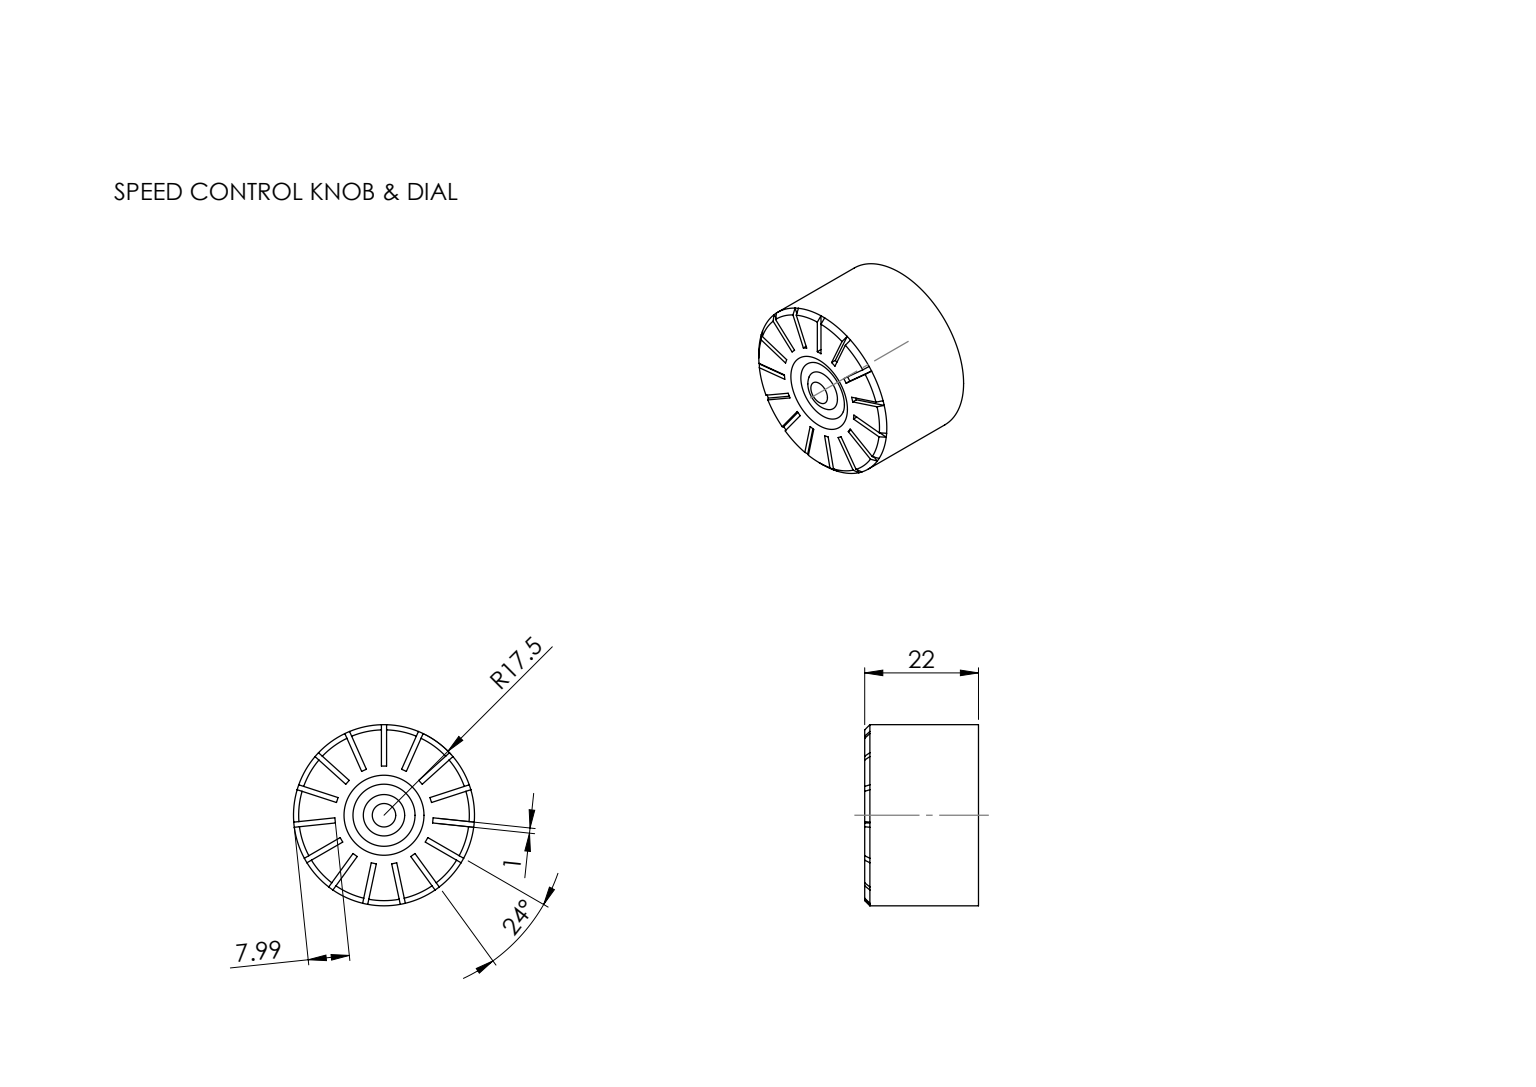
ISO-10303-21;
HEADER;
FILE_DESCRIPTION (('STEP AP214'),
    '1' );
FILE_NAME ('Speed Control Knob & Dial.step',
    '2026-10-09T15:02:13',
    ( '' ),
    ( '' ),
    'SwSTEP 2.0',
    'SolidWorks 2026',
    '' );
FILE_SCHEMA (( 'AUTOMOTIVE_DESIGN' ));
ENDSEC;

DATA;
#2=ORIENTED_EDGE ( 'NONE', *, *, #5817, .T. ) ;
#7=CARTESIAN_POINT ( 'NONE',  ( 9.881733417930924190, 8.048309972292271297, 101.0000000000000000 ) ) ;
#20=EDGE_LOOP ( 'NONE', ( #5130, #12789, #9074, #13639 ) ) ;
#24=ORIENTED_EDGE ( 'NONE', *, *, #13474, .T. ) ;
#44=DIRECTION ( 'NONE',  ( 0.000000000000000000, -0.000000000000000000, 1.000000000000000000 ) ) ;
#50=LINE ( 'NONE', #11218, #7284 ) ;
#57=ORIENTED_EDGE ( 'NONE', *, *, #15029, .T. ) ;
#62=CARTESIAN_POINT ( 'NONE',  ( -16.78599477205477797, 21.23847499609123801, 101.6666710451724214 ) ) ;
#64=CARTESIAN_POINT ( 'NONE',  ( 0.000000000000000000, 22.50000000000000000, 101.0000000000000000 ) ) ;
#65=DIRECTION ( 'NONE',  ( 0.9945218953682730678, 0.1045284632676572317, 0.000000000000000000 ) ) ;
#67=VECTOR ( 'NONE', #6603, 999.9999999999998863 ) ;
#77=ORIENTED_EDGE ( 'NONE', *, *, #283, .F. ) ;
#107=CARTESIAN_POINT ( 'NONE',  ( 0.000000000000000000, 22.50000000000000000, 102.0000000000000142 ) ) ;
#110=LINE ( 'NONE', #6455, #15051 ) ;
#112=EDGE_CURVE ( 'NONE', #12675, #13582, #5642, .T. ) ;
#127=EDGE_CURVE ( 'NONE', #6081, #8153, #2564, .T. ) ;
#131=DIRECTION ( 'NONE',  ( 0.000000000000000000, 0.000000000000000000, -1.000000000000000000 ) ) ;
#137=DIRECTION ( 'NONE',  ( 0.5000000000000039968, -0.8660254037844363761, 0.000000000000000000 ) ) ;
#142=ADVANCED_FACE ( 'NONE', ( #11706 ), #1477, .T. ) ;
#144=PLANE ( 'NONE',  #9294 ) ;
#148=PLANE ( 'NONE',  #13952 ) ;
#150=AXIS2_PLACEMENT_3D ( 'NONE', #12776, #1296, #13929 ) ;
#153=FACE_OUTER_BOUND ( 'NONE', #12318, .T. ) ;
#154=SURFACE_SIDE_STYLE ('',( #7731 ) ) ;
#162=ORIENTED_EDGE ( 'NONE', *, *, #15184, .T. ) ;
#165=ORIENTED_EDGE ( 'NONE', *, *, #12600, .T. ) ;
#166=VECTOR ( 'NONE', #9002, 1000.000000000000000 ) ;
#174=CARTESIAN_POINT ( 'NONE',  ( 14.53285685708578256, 14.68680145065703080, 102.0000000000000142 ) ) ;
#178=CIRCLE ( 'NONE', #9484, 17.50000000000000000 ) ;
#180=CARTESIAN_POINT ( 'NONE',  ( -9.189545401991425777, 24.96013318841439599, 102.0000000000000142 ) ) ;
#189=ORIENTED_EDGE ( 'NONE', *, *, #1369, .F. ) ;
#193=CARTESIAN_POINT ( 'NONE',  ( 0.000000000000000000, 22.50000000000000000, 102.0000000000000142 ) ) ;
#195=DIRECTION ( 'NONE',  ( -0.4067366430758010409, 0.9135454576426005335, 0.000000000000000000 ) ) ;
#210=EDGE_CURVE ( 'NONE', #11778, #8192, #3075, .T. ) ;
#212=CARTESIAN_POINT ( 'NONE',  ( 0.000000000000000000, 22.50000000000000000, 101.0000000000000000 ) ) ;
#224=ORIENTED_EDGE ( 'NONE', *, *, #8585, .T. ) ;
#236=PLANE ( 'NONE',  #13502 ) ;
#238=DIRECTION ( 'NONE',  ( -0.9510565162951503115, -0.3090169943749574988, 0.000000000000000000 ) ) ;
#254=CARTESIAN_POINT ( 'NONE',  ( -15.39925740754308059, 14.18658485962419569, 101.0000000000000000 ) ) ;
#264=ORIENTED_EDGE ( 'NONE', *, *, #127, .F. ) ;
#269=B_SPLINE_CURVE_WITH_KNOTS ( 'NONE', 3,
 ( #12649, #12562, #8736, #2338 ),
 .UNSPECIFIED., .F., .F.,
 ( 4, 4 ),
 ( 2.829004760667786001E-07, 0.001414802801989366570 ),
 .UNSPECIFIED. ) ;
#281=EDGE_CURVE ( 'NONE', #5931, #2031, #269, .T. ) ;
#283=EDGE_CURVE ( 'NONE', #13340, #691, #14944, .T. ) ;
#286=VERTEX_POINT ( 'NONE', #8651 ) ;
#289=FACE_OUTER_BOUND ( 'NONE', #4833, .T. ) ;
#301=DIRECTION ( 'NONE',  ( 0.9945218953682730678, 0.1045284632676572456, 0.000000000000000000 ) ) ;
#307=EDGE_CURVE ( 'NONE', #2544, #15408, #9753, .T. ) ;
#309=FACE_OUTER_BOUND ( 'NONE', #6282, .T. ) ;
#310=CARTESIAN_POINT ( 'NONE',  ( 0.000000000000000000, 22.50000000000000000, 102.0000000000000142 ) ) ;
#313=DIRECTION ( 'NONE',  ( 0.000000000000000000, 0.000000000000000000, 1.000000000000000000 ) ) ;
#322=CARTESIAN_POINT ( 'NONE',  ( -6.522576737113937817, 38.37924387995715847, 101.3333374614808662 ) ) ;
#323=ORIENTED_EDGE ( 'NONE', *, *, #16173, .F. ) ;
#325=ORIENTED_EDGE ( 'NONE', *, *, #9057, .T. ) ;
#328=CARTESIAN_POINT ( 'NONE',  ( 4.127528389677815213, 5.486372832567310454, 102.0000000000000142 ) ) ;
#337=DIRECTION ( 'NONE',  ( 1.000000000000000000, 0.000000000000000000, 0.000000000000000000 ) ) ;
#338=DIRECTION ( 'NONE',  ( 1.000000000000000000, 3.291018251567428497E-14, 0.000000000000000000 ) ) ;
#340=ADVANCED_FACE ( 'NONE', ( #12408 ), #9995, .T. ) ;
#342=DIRECTION ( 'NONE',  ( 0.000000000000000000, -0.000000000000000000, 1.000000000000000000 ) ) ;
#345=AXIS2_PLACEMENT_3D ( 'NONE', #4776, #4685, #917 ) ;
#364=ORIENTED_EDGE ( 'NONE', *, *, #5866, .F. ) ;
#367=PLANE ( 'NONE',  #5230 ) ;
#385=AXIS2_PLACEMENT_3D ( 'NONE', #4470, #15603, #705 ) ;
#387=LINE ( 'NONE', #5491, #7888 ) ;
#398=AXIS2_PLACEMENT_3D ( 'NONE', #3986, #3822, #7478 ) ;
#399=EDGE_CURVE ( 'NONE', #4332, #7924, #11576, .T. ) ;
#404=VERTEX_POINT ( 'NONE', #14726 ) ;
#413=AXIS2_PLACEMENT_3D ( 'NONE', #15842, #2171, #16155 ) ;
#414=ORIENTED_EDGE ( 'NONE', *, *, #3877, .F. ) ;
#433=ORIENTED_EDGE ( 'NONE', *, *, #9568, .T. ) ;
#446=DIRECTION ( 'NONE',  ( 0.1045284632676572456, -0.9945218953682730678, -0.000000000000000000 ) ) ;
#462=DIRECTION ( 'NONE',  ( 1.000000000000000000, 0.000000000000000000, 0.000000000000000000 ) ) ;
#474=DIRECTION ( 'NONE',  ( -0.000000000000000000, -0.000000000000000000, 1.000000000000000000 ) ) ;
#479=VECTOR ( 'NONE', #830, 1000.000000000000000 ) ;
#485=PLANE ( 'NONE',  #8421 ) ;
#502=DIRECTION ( 'NONE',  ( -0.8660254037844433705, 0.4999999999999918399, 0.000000000000000000 ) ) ;
#518=ADVANCED_FACE ( 'NONE', ( #4613 ), #3612, .F. ) ;
#544=DIRECTION ( 'NONE',  ( 1.000000000000000000, 0.000000000000000000, 0.000000000000000000 ) ) ;
#549=ORIENTED_EDGE ( 'NONE', *, *, #13824, .F. ) ;
#557=LINE ( 'NONE', #12035, #8938 ) ;
#562=VERTEX_POINT ( 'NONE', #6435 ) ;
#566=VERTEX_POINT ( 'NONE', #11495 ) ;
#569=CARTESIAN_POINT ( 'NONE',  ( 4.000000000000001776, 22.50000000000000000, 101.0000000000000000 ) ) ;
#574=DIRECTION ( 'NONE',  ( 0.000000000000000000, 0.000000000000000000, -1.000000000000000000 ) ) ;
#579=LINE ( 'NONE', #1757, #15758 ) ;
#589=VERTEX_POINT ( 'NONE', #13983 ) ;
#597=CARTESIAN_POINT ( 'NONE',  ( -8.477241335952138357, 18.18301270189218855, 101.0000000000000000 ) ) ;
#605=VERTEX_POINT ( 'NONE', #11575 ) ;
#629=AXIS2_PLACEMENT_3D ( 'NONE', #8397, #13467, #15658 ) ;
#637=CARTESIAN_POINT ( 'NONE',  ( -7.574663982647817484, 38.28367718720760138, 102.0000000000000142 ) ) ;
#646=VERTEX_POINT ( 'NONE', #3935 ) ;
#652=CARTESIAN_POINT ( 'NONE',  ( -4.056709942754369358, 5.819547430268732668, 101.3333374614808662 ) ) ;
#674=B_SPLINE_CURVE_WITH_KNOTS ( 'NONE', 3,
 ( #4274, #1766, #9418, #9340 ),
 .UNSPECIFIED., .F., .F.,
 ( 4, 4 ),
 ( 2.829004760702349710E-07, 0.001414802801989369606 ),
 .UNSPECIFIED. ) ;
#682=CARTESIAN_POINT ( 'NONE',  ( -9.877534094663211306, 8.054089844915763408, 101.0000000000000000 ) ) ;
#691=VERTEX_POINT ( 'NONE', #7507 ) ;
#694=EDGE_LOOP ( 'NONE', ( #5052, #10178, #10771, #9327 ) ) ;
#702=CARTESIAN_POINT ( 'NONE',  ( -4.127528389677584286, 5.486372832567261604, 101.0000000000000000 ) ) ;
#705=DIRECTION ( 'NONE',  ( 1.000000000000000000, 0.000000000000000000, -0.000000000000000000 ) ) ;
#707=VECTOR ( 'NONE', #13794, 1000.000000000000227 ) ;
#711=EDGE_CURVE ( 'NONE', #14691, #4152, #10547, .T. ) ;
#717=ORIENTED_EDGE ( 'NONE', *, *, #6005, .F. ) ;
#719=ORIENTED_EDGE ( 'NONE', *, *, #2125, .T. ) ;
#724=CARTESIAN_POINT ( 'NONE',  ( -4.126043002969710827, 5.493361027597350343, 101.0000000000000000 ) ) ;
#729=DIRECTION ( 'NONE',  ( -0.000000000000000000, -0.000000000000000000, 1.000000000000000000 ) ) ;
#731=CARTESIAN_POINT ( 'NONE',  ( 6.661118525004998681, 38.69041383028350367, 102.0000000000000142 ) ) ;
#734=FACE_OUTER_BOUND ( 'NONE', #14301, .T. ) ;
#739=ORIENTED_EDGE ( 'NONE', *, *, #10784, .T. ) ;
#742=LINE ( 'NONE', #7236, #3369 ) ;
#744=ORIENTED_EDGE ( 'NONE', *, *, #13835, .F. ) ;
#760=EDGE_CURVE ( 'NONE', #1819, #7317, #14134, .T. ) ;
#769=CARTESIAN_POINT ( 'NONE',  ( 0.000000000000000000, 22.50000000000000000, 101.0000000000000000 ) ) ;
#778=ORIENTED_EDGE ( 'NONE', *, *, #1765, .T. ) ;
#792=LINE ( 'NONE', #5882, #7783 ) ;
#793=VERTEX_POINT ( 'NONE', #6609 ) ;
#794=EDGE_CURVE ( 'NONE', #9739, #6366, #6691, .T. ) ;
#797=ORIENTED_EDGE ( 'NONE', *, *, #14711, .F. ) ;
#800=EDGE_CURVE ( 'NONE', #6081, #8593, #7999, .T. ) ;
#818=ORIENTED_EDGE ( 'NONE', *, *, #5743, .T. ) ;
#828=DIRECTION ( 'NONE',  ( 1.000000000000000000, -5.352861011585576290E-15, 0.000000000000000000 ) ) ;
#830=DIRECTION ( 'NONE',  ( -0.000000000000000000, -0.000000000000000000, 1.000000000000000000 ) ) ;
#833=LINE ( 'NONE', #15967, #10244 ) ;
#836=CARTESIAN_POINT ( 'NONE',  ( 0.000000000000000000, 22.50000000000000000, 80.00000000000000000 ) ) ;
#845=DIRECTION ( 'NONE',  ( -0.9135454576426004225, -0.4067366430758009854, 0.000000000000000000 ) ) ;
#860=VERTEX_POINT ( 'NONE', #11908 ) ;
#874=CARTESIAN_POINT ( 'NONE',  ( 3.407225380398686276, 31.38205016914263723, 102.0000000000000142 ) ) ;
#875=ORIENTED_EDGE ( 'NONE', *, *, #8946, .T. ) ;
#878=DIRECTION ( 'NONE',  ( 0.8660254037844363761, 0.5000000000000041078, 0.000000000000000000 ) ) ;
#888=CARTESIAN_POINT ( 'NONE',  ( -6.661118525005218949, 38.69041383028340420, 102.0000000000000142 ) ) ;
#889=DIRECTION ( 'NONE',  ( -0.000000000000000000, -0.000000000000000000, 1.000000000000000000 ) ) ;
#890=DIRECTION ( 'NONE',  ( 0.000000000000000000, 0.000000000000000000, -1.000000000000000000 ) ) ;
#895=VERTEX_POINT ( 'NONE', #1676 ) ;
#900=ORIENTED_EDGE ( 'NONE', *, *, #11699, .F. ) ;
#915=EDGE_CURVE ( 'NONE', #9440, #646, #6307, .T. ) ;
#917=DIRECTION ( 'NONE',  ( 1.000000000000000000, 0.000000000000000000, 0.000000000000000000 ) ) ;
#918=ORIENTED_EDGE ( 'NONE', *, *, #1112, .T. ) ;
#919=DIRECTION ( 'NONE',  ( -0.000000000000000000, 0.000000000000000000, 1.000000000000000000 ) ) ;
#925=DIRECTION ( 'NONE',  ( -0.000000000000000000, -0.000000000000000000, -1.000000000000000000 ) ) ;
#926=LINE ( 'NONE', #8666, #14148 ) ;
#927=DIRECTION ( 'NONE',  ( 0.000000000000000000, 0.000000000000000000, 1.000000000000000000 ) ) ;
#941=ORIENTED_EDGE ( 'NONE', *, *, #4990, .F. ) ;
#956=VECTOR ( 'NONE', #12319, 1000.000000000000000 ) ;
#959=ORIENTED_EDGE ( 'NONE', *, *, #281, .F. ) ;
#960=VERTEX_POINT ( 'NONE', #8246 ) ;
#977=ORIENTED_EDGE ( 'NONE', *, *, #9370, .T. ) ;
#987=( NAMED_UNIT ( * ) PLANE_ANGLE_UNIT ( ) SI_UNIT ( $, .RADIAN. ) );
#989=CARTESIAN_POINT ( 'NONE',  ( -16.16503364901097939, 28.27806893495044349, 101.3333374614808662 ) ) ;
#996=CARTESIAN_POINT ( 'NONE',  ( 0.000000000000000000, 22.50000000000000000, 101.0000000000000000 ) ) ;
#1002=EDGE_CURVE ( 'NONE', #11153, #15748, #13312, .T. ) ;
#1005=LINE ( 'NONE', #8661, #11852 ) ;
#1007=CARTESIAN_POINT ( 'NONE',  ( 14.61046079763427130, 13.48729625631194118, 101.3333374614808662 ) ) ;
#1033=ADVANCED_FACE ( 'NONE', ( #14549 ), #10907, .F. ) ;
#1037=ADVANCED_FACE ( 'NONE', ( #12061 ), #4680, .T. ) ;
#1040=EDGE_LOOP ( 'NONE', ( #13375, #11613, #1901, #5104 ) ) ;
#1041=ORIENTED_EDGE ( 'NONE', *, *, #14423, .T. ) ;
#1044=LINE ( 'NONE', #12452, #15798 ) ;
#1047=CIRCLE ( 'NONE', #1583, 2.267949192431125027 ) ;
#1052=CARTESIAN_POINT ( 'NONE',  ( -15.53071739328007794, 28.07196708982276334, 102.0000000000000142 ) ) ;
#1054=FACE_OUTER_BOUND ( 'NONE', #13700, .T. ) ;
#1057=EDGE_LOOP ( 'NONE', ( #1893, #7443, #15977, #14426 ) ) ;
#1083=VERTEX_POINT ( 'NONE', #4517 ) ;
#1085=ORIENTED_EDGE ( 'NONE', *, *, #15147, .F. ) ;
#1086=DIRECTION ( 'NONE',  ( -0.8660254037844433705, 0.4999999999999918954, 0.000000000000000000 ) ) ;
#1094=PLANE ( 'NONE',  #12119 ) ;
#1100=EDGE_CURVE ( 'NONE', #1499, #2544, #12417, .T. ) ;
#1101=VERTEX_POINT ( 'NONE', #7092 ) ;
#1109=ADVANCED_FACE ( 'NONE', ( #13477 ), #12152, .T. ) ;
#1112=EDGE_CURVE ( 'NONE', #860, #7211, #5048, .T. ) ;
#1115=ADVANCED_FACE ( 'NONE', ( #1155 ), #12485, .T. ) ;
#1118=ORIENTED_EDGE ( 'NONE', *, *, #15652, .T. ) ;
#1123=CARTESIAN_POINT ( 'NONE',  ( 17.44929222242216227, 21.16875962481693207, 101.0000000000000000 ) ) ;
#1125=DIRECTION ( 'NONE',  ( 0.000000000000000000, 0.000000000000000000, -1.000000000000000000 ) ) ;
#1130=CARTESIAN_POINT ( 'NONE',  ( 4.320770838041294581, 30.97531352606685218, 101.0000000000000000 ) ) ;
#1134=ORIENTED_EDGE ( 'NONE', *, *, #1002, .F. ) ;
#1139=ADVANCED_FACE ( 'NONE', ( #16220 ), #10024, .T. ) ;
#1141=LINE ( 'NONE', #8801, #3640 ) ;
#1145=ORIENTED_EDGE ( 'NONE', *, *, #1475, .F. ) ;
#1148=CARTESIAN_POINT ( 'NONE',  ( 0.000000000000000000, 22.50000000000000000, 102.0000000000000142 ) ) ;
#1151=DIRECTION ( 'NONE',  ( 0.8660254037844432595, -0.4999999999999920064, 0.000000000000000000 ) ) ;
#1155=FACE_OUTER_BOUND ( 'NONE', #4460, .T. ) ;
#1161=EDGE_LOOP ( 'NONE', ( #1118, #2203, #12678, #13882 ) ) ;
#1168=DIRECTION ( 'NONE',  ( 0.000000000000000000, 0.000000000000000000, -1.000000000000000000 ) ) ;
#1182=AXIS2_PLACEMENT_3D ( 'NONE', #5912, #10972, #15193 ) ;
#1200=ORIENTED_EDGE ( 'NONE', *, *, #13732, .F. ) ;
#1201=AXIS2_PLACEMENT_3D ( 'NONE', #11274, #16332, #1361 ) ;
#1208=CARTESIAN_POINT ( 'NONE',  ( 1.486087262401875941, 13.10364194761998213, 101.0000000000000000 ) ) ;
#1218=DIRECTION ( 'NONE',  ( 0.000000000000000000, 0.000000000000000000, -1.000000000000000000 ) ) ;
#1219=CIRCLE ( 'NONE', #2556, 16.50000000000000711 ) ;
#1221=EDGE_CURVE ( 'NONE', #14428, #404, #5255, .T. ) ;
#1233=AXIS2_PLACEMENT_3D ( 'NONE', #15547, #11894, #4178 ) ;
#1237=CARTESIAN_POINT ( 'NONE',  ( 0.000000000000000000, 22.50000000000000000, 102.0000000000000142 ) ) ;
#1239=CARTESIAN_POINT ( 'NONE',  ( 0.000000000000000000, 22.50000000000000000, 102.0000000000000142 ) ) ;
#1246=DIRECTION ( 'NONE',  ( 0.000000000000000000, 0.000000000000000000, -1.000000000000000000 ) ) ;
#1249=EDGE_LOOP ( 'NONE', ( #3388, #224, #10891, #15269 ) ) ;
#1250=EDGE_CURVE ( 'NONE', #9378, #8439, #5819, .T. ) ;
#1251=CARTESIAN_POINT ( 'NONE',  ( 0.000000000000000000, 22.50000000000000000, 101.0000000000000000 ) ) ;
#1252=ORIENTED_EDGE ( 'NONE', *, *, #15652, .F. ) ;
#1262=LINE ( 'NONE', #8827, #166 ) ;
#1264=DIRECTION ( 'NONE',  ( 1.000000000000000000, 0.000000000000000000, 0.000000000000000000 ) ) ;
#1266=CARTESIAN_POINT ( 'NONE',  ( 0.000000000000000000, 22.50000000000000000, 101.0000000000000000 ) ) ;
#1271=EDGE_CURVE ( 'NONE', #1479, #2396, #6753, .T. ) ;
#1276=ORIENTED_EDGE ( 'NONE', *, *, #15012, .T. ) ;
#1291=EDGE_LOOP ( 'NONE', ( #5186, #12830, #15543, #6502 ) ) ;
#1296=DIRECTION ( 'NONE',  ( 0.000000000000000000, 0.000000000000000000, -1.000000000000000000 ) ) ;
#1305=ORIENTED_EDGE ( 'NONE', *, *, #14153, .F. ) ;
#1310=ORIENTED_EDGE ( 'NONE', *, *, #14892, .T. ) ;
#1319=CARTESIAN_POINT ( 'NONE',  ( 7.394441145214595501, 28.48516834767053751, 101.0000000000000000 ) ) ;
#1326=VERTEX_POINT ( 'NONE', #11799 ) ;
#1331=CARTESIAN_POINT ( 'NONE',  ( -4.127528389677584286, 5.486372832567261604, 101.0000000000000000 ) ) ;
#1336=CARTESIAN_POINT ( 'NONE',  ( -10.69075041230567891, 8.636095224584611429, 101.0000000000000000 ) ) ;
#1354=EDGE_CURVE ( 'NONE', #13340, #7372, #2628, .T. ) ;
#1361=DIRECTION ( 'NONE',  ( -1.000000000000000000, 0.000000000000000000, 0.000000000000000000 ) ) ;
#1369=EDGE_CURVE ( 'NONE', #9016, #14108, #178, .T. ) ;
#1372=ORIENTED_EDGE ( 'NONE', *, *, #7951, .F. ) ;
#1376=ADVANCED_FACE ( 'NONE', ( #9478 ), #8468, .F. ) ;
#1384=LINE ( 'NONE', #16276, #6059 ) ;
#1389=ORIENTED_EDGE ( 'NONE', *, *, #1354, .F. ) ;
#1393=DIRECTION ( 'NONE',  ( -0.3090169943749573878, 0.9510565162951503115, 0.000000000000000000 ) ) ;
#1396=DIRECTION ( 'NONE',  ( -0.7431448254773861395, -0.6691306063588672304, 0.000000000000000000 ) ) ;
#1398=DIRECTION ( 'NONE',  ( 0.8090169943749504489, -0.5877852522924689183, 0.000000000000000000 ) ) ;
#1404=CARTESIAN_POINT ( 'NONE',  ( 1.486087262401875941, 13.10364194761998213, 101.0000000000000000 ) ) ;
#1412=CARTESIAN_POINT ( 'NONE',  ( 0.000000000000000000, 22.50000000000000000, 102.0000000000000142 ) ) ;
#1433=ORIENTED_EDGE ( 'NONE', *, *, #15400, .T. ) ;
#1451=AXIS2_PLACEMENT_3D ( 'NONE', #6325, #11391, #3740 ) ;
#1458=VECTOR ( 'NONE', #4886, 999.9999999999998863 ) ;
#1466=LINE ( 'NONE', #4050, #4788 ) ;
#1470=DIRECTION ( 'NONE',  ( 1.224646799147353207E-16, 1.000000000000000000, -0.000000000000000000 ) ) ;
#1475=EDGE_CURVE ( 'NONE', #14428, #7907, #7062, .T. ) ;
#1476=ORIENTED_EDGE ( 'NONE', *, *, #12004, .T. ) ;
#1477=PLANE ( 'NONE',  #14226 ) ;
#1479=VERTEX_POINT ( 'NONE', #8774 ) ;
#1482=CARTESIAN_POINT ( 'NONE',  ( 7.300484685132999196, 37.66786040234666189, 101.6666710451724214 ) ) ;
#1485=VECTOR ( 'NONE', #16302, 1000.000000000000000 ) ;
#1487=AXIS2_PLACEMENT_3D ( 'NONE', #7913, #11658, #14139 ) ;
#1495=DIRECTION ( 'NONE',  ( -0.3090169943749574988, 0.9510565162951503115, 0.000000000000000000 ) ) ;
#1497=CARTESIAN_POINT ( 'NONE',  ( 15.83973438765496056, 27.12091057352781931, 102.0000000000000142 ) ) ;
#1499=VERTEX_POINT ( 'NONE', #14772 ) ;
#1511=LINE ( 'NONE', #10413, #67 ) ;
#1515=VECTOR ( 'NONE', #9722, 1000.000000000000000 ) ;
#1524=ADVANCED_FACE ( 'NONE', ( #5735 ), #9807, .T. ) ;
#1527=EDGE_CURVE ( 'NONE', #3819, #3901, #12127, .T. ) ;
#1533=B_SPLINE_CURVE_WITH_KNOTS ( 'NONE', 3,
 ( #5559, #2707, #9037, #14261 ),
 .UNSPECIFIED., .F., .F.,
 ( 4, 4 ),
 ( 2.829004760673920638E-07, 0.001414802801989365486 ),
 .UNSPECIFIED. ) ;
#1537=LINE ( 'NONE', #6373, #11863 ) ;
#1547=ORIENTED_EDGE ( 'NONE', *, *, #15147, .T. ) ;
#1548=CARTESIAN_POINT ( 'NONE',  ( -13.22516817658079624, 40.70288237343621063, 101.0000000000000000 ) ) ;
#1550=CARTESIAN_POINT ( 'NONE',  ( -14.82166083077704499, 14.52006039870307852, 101.6666710451724214 ) ) ;
#1558=FACE_OUTER_BOUND ( 'NONE', #10631, .T. ) ;
#1561=ORIENTED_EDGE ( 'NONE', *, *, #11744, .T. ) ;
#1562=CARTESIAN_POINT ( 'NONE',  ( -0.5000000000000000000, 39.65938208326293335, 101.3333374618097480 ) ) ;
#1563=EDGE_LOOP ( 'NONE', ( #13749, #13457, #3721, #959 ) ) ;
#1564=ORIENTED_EDGE ( 'NONE', *, *, #1250, .T. ) ;
#1570=VECTOR ( 'NONE', #9716, 1000.000000000000114 ) ;
#1573=DIRECTION ( 'NONE',  ( -0.000000000000000000, -0.000000000000000000, 1.000000000000000000 ) ) ;
#1583=AXIS2_PLACEMENT_3D ( 'NONE', #310, #15194, #13947 ) ;
#1584=ORIENTED_EDGE ( 'NONE', *, *, #1798, .F. ) ;
#1593=CARTESIAN_POINT ( 'NONE',  ( 0.000000000000000000, 22.50000000000000000, 102.0000000000000142 ) ) ;
#1601=FACE_OUTER_BOUND ( 'NONE', #8159, .T. ) ;
#1622=EDGE_LOOP ( 'NONE', ( #5422, #797, #7323, #9730 ) ) ;
#1635=CARTESIAN_POINT ( 'NONE',  ( -6.725310538855818976, 29.22831317314782851, 101.0000000000000000 ) ) ;
#1636=ORIENTED_EDGE ( 'NONE', *, *, #16217, .T. ) ;
#1641=VERTEX_POINT ( 'NONE', #2989 ) ;
#1656=FACE_OUTER_BOUND ( 'NONE', #3657, .T. ) ;
#1660=ORIENTED_EDGE ( 'NONE', *, *, #5200, .T. ) ;
#1662=ADVANCED_FACE ( 'NONE', ( #1656 ), #485, .T. ) ;
#1674=CARTESIAN_POINT ( 'NONE',  ( 5.988468393966018155, 15.10823117958429584, 101.0000000000000000 ) ) ;
#1676=CARTESIAN_POINT ( 'NONE',  ( -2.464234863135557063, 13.31155363843772932, 102.0000000000000142 ) ) ;
#1685=ORIENTED_EDGE ( 'NONE', *, *, #6952, .T. ) ;
#1702=ORIENTED_EDGE ( 'NONE', *, *, #5817, .F. ) ;
#1705=CARTESIAN_POINT ( 'NONE',  ( -17.35186893731094671, 20.17349094513186358, 101.0000000000000000 ) ) ;
#1726=DIRECTION ( 'NONE',  ( 0.000000000000000000, 0.000000000000000000, -1.000000000000000000 ) ) ;
#1735=CIRCLE ( 'NONE', #12622, 4.000000000000001776 ) ;
#1736=DIRECTION ( 'NONE',  ( 0.5000000000000039968, -0.8660254037844363761, 0.000000000000000000 ) ) ;
#1744=AXIS2_PLACEMENT_3D ( 'NONE', #14955, #16212, #4844 ) ;
#1747=VECTOR ( 'NONE', #4128, 1000.000000000000000 ) ;
#1757=CARTESIAN_POINT ( 'NONE',  ( 0.5000000000000000000, 39.99999999999999289, 102.0000000000000142 ) ) ;
#1762=CIRCLE ( 'NONE', #5243, 17.50000000000000000 ) ;
#1765=EDGE_CURVE ( 'NONE', #5661, #2974, #3228, .T. ) ;
#1766=CARTESIAN_POINT ( 'NONE',  ( 13.08647130699016614, 33.61029532559867050, 101.3333374614808662 ) ) ;
#1769=VERTEX_POINT ( 'NONE', #13455 ) ;
#1770=CARTESIAN_POINT ( 'NONE',  ( 0.000000000000000000, 22.50000000000000000, 101.0000000000000000 ) ) ;
#1772=VECTOR ( 'NONE', #11819, 1000.000000000000000 ) ;
#1775=VECTOR ( 'NONE', #15211, 1000.000000000000000 ) ;
#1779=DIRECTION ( 'NONE',  ( 0.9945218953682730678, 0.1045284632676572456, 0.000000000000000000 ) ) ;
#1790=ORIENTED_EDGE ( 'NONE', *, *, #2785, .T. ) ;
#1791=LINE ( 'NONE', #13102, #1747 ) ;
#1795=DIRECTION ( 'NONE',  ( -0.7431448254773954654, 0.6691306063588569053, 0.000000000000000000 ) ) ;
#1798=EDGE_CURVE ( 'NONE', #13034, #9095, #2062, .T. ) ;
#1819=VERTEX_POINT ( 'NONE', #7313 ) ;
#1822=ORIENTED_EDGE ( 'NONE', *, *, #13766, .T. ) ;
#1826=ORIENTED_EDGE ( 'NONE', *, *, #1221, .T. ) ;
#1827=CARTESIAN_POINT ( 'NONE',  ( -10.09851121871618140, 9.451242543235633065, 102.0000000000000142 ) ) ;
#1831=ADVANCED_FACE ( 'NONE', ( #734 ), #8442, .T. ) ;
#1836=CARTESIAN_POINT ( 'NONE',  ( 3.147895402236133400, 5.285449336779636909, 101.0000000000000000 ) ) ;
#1841=EDGE_CURVE ( 'NONE', #7924, #286, #1384, .T. ) ;
#1859=ADVANCED_FACE ( 'NONE', ( #12864 ), #16446, .F. ) ;
#1864=FACE_OUTER_BOUND ( 'NONE', #13111, .T. ) ;
#1873=EDGE_CURVE ( 'NONE', #2880, #10320, #13746, .T. ) ;
#1893=ORIENTED_EDGE ( 'NONE', *, *, #1112, .F. ) ;
#1897=ORIENTED_EDGE ( 'NONE', *, *, #13064, .F. ) ;
#1901=ORIENTED_EDGE ( 'NONE', *, *, #5685, .F. ) ;
#1903=CARTESIAN_POINT ( 'NONE',  ( -3.918041248536338728, 6.471932344328960696, 102.0000000000000142 ) ) ;
#1918=UNCERTAINTY_MEASURE_WITH_UNIT (LENGTH_MEASURE( 1.000000000000000082E-05 ), #12798, 'distance_accuracy_value', 'NONE');
#1921=CARTESIAN_POINT ( 'NONE',  ( 14.90544456622775904, 13.31698729810792692, 101.0000000000000000 ) ) ;
#1929=DIRECTION ( 'NONE',  ( 0.4067366430758010964, -0.9135454576426004225, 0.000000000000000000 ) ) ;
#1932=VECTOR ( 'NONE', #15469, 999.9999999999998863 ) ;
#1944=ORIENTED_EDGE ( 'NONE', *, *, #5416, .F. ) ;
#1945=CARTESIAN_POINT ( 'NONE',  ( 3.918041248536554555, 6.471932344329013098, 102.0000000000000142 ) ) ;
#1948=CARTESIAN_POINT ( 'NONE',  ( 0.000000000000000000, 22.50000000000000000, 102.0000000000000142 ) ) ;
#1991=DIRECTION ( 'NONE',  ( 0.000000000000000000, 0.000000000000000000, -1.000000000000000000 ) ) ;
#2002=VECTOR ( 'NONE', #16137, 1000.000000000000000 ) ;
#2015=VECTOR ( 'NONE', #7830, 1000.000000000000000 ) ;
#2017=FACE_OUTER_BOUND ( 'NONE', #8126, .T. ) ;
#2031=VERTEX_POINT ( 'NONE', #12201 ) ;
#2039=VECTOR ( 'NONE', #16120, 1000.000000000000114 ) ;
#2046=ADVANCED_FACE ( 'NONE', ( #9713 ), #3396, .F. ) ;
#2060=CARTESIAN_POINT ( 'NONE',  ( 15.83973438765496056, 27.12091057352781931, 102.0000000000000142 ) ) ;
#2062=LINE ( 'NONE', #8382, #3390 ) ;
#2063=CARTESIAN_POINT ( 'NONE',  ( -7.571758127758879908, 38.27715053026740577, 101.0000000000000000 ) ) ;
#2068=ORIENTED_EDGE ( 'NONE', *, *, #7249, .T. ) ;
#2076=DIRECTION ( 'NONE',  ( 0.000000000000000000, 0.000000000000000000, -1.000000000000000000 ) ) ;
#2079=DIRECTION ( 'NONE',  ( 1.000000000000000000, 7.930164461608261426E-16, 0.000000000000000000 ) ) ;
#2088=PRODUCT_DEFINITION_CONTEXT ( 'detailed design', #14591, 'design' ) ;
#2093=FACE_OUTER_BOUND ( 'NONE', #8210, .T. ) ;
#2096=STYLED_ITEM ( 'NONE', ( #12300 ), #3320 ) ;
#2114=LINE ( 'NONE', #5876, #1458 ) ;
#2125=EDGE_CURVE ( 'NONE', #404, #7781, #14519, .T. ) ;
#2126=ORIENTED_EDGE ( 'NONE', *, *, #13766, .F. ) ;
#2140=CARTESIAN_POINT ( 'NONE',  ( -0.4999999999999990563, 31.99999999999998579, 101.0000000000000000 ) ) ;
#2146=ORIENTED_EDGE ( 'NONE', *, *, #10006, .T. ) ;
#2150=ORIENTED_EDGE ( 'NONE', *, *, #15029, .F. ) ;
#2152=DIRECTION ( 'NONE',  ( 0.5877852522924688072, 0.8090169943749505599, 0.000000000000000000 ) ) ;
#2158=CARTESIAN_POINT ( 'NONE',  ( 0.000000000000000000, 0.000000000000000000, 0.000000000000000000 ) ) ;
#2164=DIRECTION ( 'NONE',  ( 1.000000000000000000, 0.000000000000000000, 0.000000000000000000 ) ) ;
#2166=CARTESIAN_POINT ( 'NONE',  ( 9.485510086921706829, 8.593664601562213790, 101.6666710451724214 ) ) ;
#2169=LINE ( 'NONE', #12241, #956 ) ;
#2171=DIRECTION ( 'NONE',  ( -0.3090169943749448422, -0.9510565162951544194, 0.000000000000000000 ) ) ;
#2188=ORIENTED_EDGE ( 'NONE', *, *, #9653, .T. ) ;
#2203=ORIENTED_EDGE ( 'NONE', *, *, #13732, .T. ) ;
#2207=CARTESIAN_POINT ( 'NONE',  ( 12.16951863902660236, 34.13030016454095517, 101.6666710451724214 ) ) ;
#2224=VERTEX_POINT ( 'NONE', #2382 ) ;
#2229=DIRECTION ( 'NONE',  ( 0.000000000000000000, 1.000000000000000000, 0.000000000000000000 ) ) ;
#2236=CARTESIAN_POINT ( 'NONE',  ( -15.84787772126911776, 28.17501872725009093, 101.6666710451724214 ) ) ;
#2238=DIRECTION ( 'NONE',  ( 0.8090169943749426773, 0.5877852522924797984, 0.000000000000000000 ) ) ;
#2249=CARTESIAN_POINT ( 'NONE',  ( 9.681523229999685398, 8.323875655254958872, 101.3333374614808662 ) ) ;
#2253=VECTOR ( 'NONE', #11449, 1000.000000000000114 ) ;
#2254=EDGE_CURVE ( 'NONE', #7234, #12941, #8612, .T. ) ;
#2263=EDGE_CURVE ( 'NONE', #5800, #1641, #12454, .T. ) ;
#2267=AXIS2_PLACEMENT_3D ( 'NONE', #7, #12739, #12815 ) ;
#2277=VECTOR ( 'NONE', #16147, 1000.000000000000000 ) ;
#2280=CIRCLE ( 'NONE', #5231, 17.50000000000000000 ) ;
#2292=CARTESIAN_POINT ( 'NONE',  ( -8.880528407616480990, 25.91118970470954963, 101.0000000000000000 ) ) ;
#2293=ORIENTED_EDGE ( 'NONE', *, *, #6374, .T. ) ;
#2297=CARTESIAN_POINT ( 'NONE',  ( -3.407225380398804404, 31.38205016914259105, 102.0000000000000142 ) ) ;
#2301=ADVANCED_FACE ( 'NONE', ( #4900 ), #15014, .F. ) ;
#2309=CIRCLE ( 'NONE', #14787, 6.000000000000001776 ) ;
#2316=ORIENTED_EDGE ( 'NONE', *, *, #14670, .T. ) ;
#2322=DIRECTION ( 'NONE',  ( -0.000000000000000000, 0.000000000000000000, 1.000000000000000000 ) ) ;
#2323=LINE ( 'NONE', #5260, #14851 ) ;
#2325=CARTESIAN_POINT ( 'NONE',  ( -15.53071739328007794, 28.07196708982276334, 102.0000000000000142 ) ) ;
#2338=CARTESIAN_POINT ( 'NONE',  ( -14.03285685708567065, 13.82077604687239258, 102.0000000000000142 ) ) ;
#2347=CARTESIAN_POINT ( 'NONE',  ( 13.22516817658054933, 40.70288237343638826, 101.0000000000000000 ) ) ;
#2352=PLANE ( 'NONE',  #5274 ) ;
#2358=EDGE_CURVE ( 'NONE', #15408, #2396, #13233, .T. ) ;
#2375=DIRECTION ( 'NONE',  ( -0.000000000000000000, -0.000000000000000000, 1.000000000000000000 ) ) ;
#2377=ORIENTED_EDGE ( 'NONE', *, *, #14727, .T. ) ;
#2382=CARTESIAN_POINT ( 'NONE',  ( 9.189545401991395579, 24.96013318841451678, 102.0000000000000142 ) ) ;
#2391=EDGE_CURVE ( 'NONE', #3858, #9016, #6881, .T. ) ;
#2396=VERTEX_POINT ( 'NONE', #12147 ) ;
#2401=ORIENTED_EDGE ( 'NONE', *, *, #794, .T. ) ;
#2411=CARTESIAN_POINT ( 'NONE',  ( 6.251299836021209089, 37.76994598419266680, 102.0000000000000142 ) ) ;
#2416=ORIENTED_EDGE ( 'NONE', *, *, #15170, .F. ) ;
#2422=LINE ( 'NONE', #13734, #11051 ) ;
#2459=FACE_OUTER_BOUND ( 'NONE', #4151, .T. ) ;
#2467=CARTESIAN_POINT ( 'NONE',  ( -7.571758127758879908, 38.27715053026740577, 101.0000000000000000 ) ) ;
#2468=EDGE_CURVE ( 'NONE', #7372, #2224, #3246, .T. ) ;
#2471=DIRECTION ( 'NONE',  ( 1.000000000000000000, 0.000000000000000000, 0.000000000000000000 ) ) ;
#2481=VECTOR ( 'NONE', #13307, 1000.000000000000000 ) ;
#2485=DIRECTION ( 'NONE',  ( 1.000000000000000000, 0.000000000000000000, 0.000000000000000000 ) ) ;
#2488=FACE_OUTER_BOUND ( 'NONE', #20, .T. ) ;
#2492=DIRECTION ( 'NONE',  ( 0.2079116908177664202, -0.9781476007338041345, 0.000000000000000000 ) ) ;
#2505=AXIS2_PLACEMENT_3D ( 'NONE', #14076, #2691, #3785 ) ;
#2540=ORIENTED_EDGE ( 'NONE', *, *, #9370, .F. ) ;
#2544=VERTEX_POINT ( 'NONE', #13551 ) ;
#2546=LINE ( 'NONE', #2297, #2253 ) ;
#2548=CARTESIAN_POINT ( 'NONE',  ( -7.977241335952133916, 17.31698729810774751, 101.0000000000000000 ) ) ;
#2553=CIRCLE ( 'NONE', #13434, 17.50000000000000000 ) ;
#2556=AXIS2_PLACEMENT_3D ( 'NONE', #1237, #3744, #6331 ) ;
#2557=ADVANCED_FACE ( 'NONE', ( #11071 ), #4767, .T. ) ;
#2558=DIRECTION ( 'NONE',  ( -0.5877852522924797984, 0.8090169943749424553, 0.000000000000000000 ) ) ;
#2564=LINE ( 'NONE', #7643, #8117 ) ;
#2568=DIRECTION ( 'NONE',  ( 0.000000000000000000, -0.000000000000000000, -1.000000000000000000 ) ) ;
#2572=CARTESIAN_POINT ( 'NONE',  ( 0.000000000000000000, 22.50000000000000000, 101.0000000000000000 ) ) ;
#2580=DIRECTION ( 'NONE',  ( 0.9781476007338041345, 0.2079116908177664202, 0.000000000000000000 ) ) ;
#2585=ORIENTED_EDGE ( 'NONE', *, *, #16278, .T. ) ;
#2590=LINE ( 'NONE', #12895, #1775 ) ;
#2596=DIRECTION ( 'NONE',  ( -0.9945218953682744001, 0.1045284632676435205, 0.000000000000000000 ) ) ;
#2598=EDGE_CURVE ( 'NONE', #8439, #16202, #5043, .T. ) ;
#2606=AXIS2_PLACEMENT_3D ( 'NONE', #5818, #131, #5078 ) ;
#2614=FACE_OUTER_BOUND ( 'NONE', #8305, .T. ) ;
#2617=AXIS2_PLACEMENT_3D ( 'NONE', #12532, #1125, #15100 ) ;
#2628=B_SPLINE_CURVE_WITH_KNOTS ( 'NONE', 3,
 ( #2987, #8056, #2736, #1497 ),
 .UNSPECIFIED., .F., .F.,
 ( 4, 4 ),
 ( 2.829004760679149478E-07, 0.001414802801989369172 ),
 .UNSPECIFIED. ) ;
#2629=CARTESIAN_POINT ( 'NONE',  ( -12.16951863902676223, 34.13030016454078464, 101.6666710451724214 ) ) ;
#2640=ORIENTED_EDGE ( 'NONE', *, *, #9573, .F. ) ;
#2648=CARTESIAN_POINT ( 'NONE',  ( 0.5000000000000009992, 31.99999999999998579, 101.0000000000000000 ) ) ;
#2649=CARTESIAN_POINT ( 'NONE',  ( 2.464234863135679188, 13.31155363843775064, 102.0000000000000142 ) ) ;
#2651=EDGE_CURVE ( 'NONE', #15408, #1769, #15198, .T. ) ;
#2654=CARTESIAN_POINT ( 'NONE',  ( -5.988468393965924008, 15.10823117958422301, 102.0000000000000142 ) ) ;
#2655=DIRECTION ( 'NONE',  ( 0.8090169943749505599, -0.5877852522924688072, -0.000000000000000000 ) ) ;
#2660=DIRECTION ( 'NONE',  ( 0.000000000000000000, 0.000000000000000000, -1.000000000000000000 ) ) ;
#2663=CARTESIAN_POINT ( 'NONE',  ( -6.658212670116278709, 38.68388717334321569, 101.0000000000000000 ) ) ;
#2664=VERTEX_POINT ( 'NONE', #7730 ) ;
#2685=ORIENTED_EDGE ( 'NONE', *, *, #12100, .T. ) ;
#2691=DIRECTION ( 'NONE',  ( 0.9781476007338041345, 0.2079116908177665313, 0.000000000000000000 ) ) ;
#2698=ADVANCED_FACE ( 'NONE', ( #153 ), #3746, .T. ) ;
#2706=DIRECTION ( 'NONE',  ( 0.9945218953682730678, 0.1045284632676572317, 0.000000000000000000 ) ) ;
#2707=CARTESIAN_POINT ( 'NONE',  ( 15.11046079763426420, 14.35332166009638222, 101.3333374614808662 ) ) ;
#2718=AXIS2_PLACEMENT_3D ( 'NONE', #10721, #12040, #4408 ) ;
#2723=ORIENTED_EDGE ( 'NONE', *, *, #4292, .F. ) ;
#2729=DIRECTION ( 'NONE',  ( -0.000000000000000000, -0.000000000000000000, -1.000000000000000000 ) ) ;
#2733=VECTOR ( 'NONE', #7619, 1000.000000000000000 ) ;
#2736=CARTESIAN_POINT ( 'NONE',  ( 16.15689471564400037, 27.22396221095515045, 101.6666710451724214 ) ) ;
#2740=PRODUCT_DEFINITION ( 'UNKNOWN', '', #6278, #2088 ) ;
#2743=VERTEX_POINT ( 'NONE', #14364 ) ;
#2752=LINE ( 'NONE', #3085, #16275 ) ;
#2779=DIRECTION ( 'NONE',  ( -0.9945218953682744001, 0.1045284632676435205, 0.000000000000000000 ) ) ;
#2785=EDGE_CURVE ( 'NONE', #10405, #10911, #9472, .T. ) ;
#2793=CARTESIAN_POINT ( 'NONE',  ( -15.39925740754308059, 14.18658485962419569, 101.0000000000000000 ) ) ;
#2808=CARTESIAN_POINT ( 'NONE',  ( -0.5000000000000000000, 39.99285568453590400, 101.0000000000000000 ) ) ;
#2809=EDGE_LOOP ( 'NONE', ( #5254, #6057, #13537, #8063 ) ) ;
#2819=CONICAL_SURFACE ( 'NONE', #3355, 16.50000000000000711, 0.7853981633974447263 ) ;
#2826=CARTESIAN_POINT ( 'NONE',  ( -5.988468393965924008, 15.10823117958422301, 101.0000000000000000 ) ) ;
#2834=VECTOR ( 'NONE', #14855, 1000.000000000000000 ) ;
#2837=DIRECTION ( 'NONE',  ( -0.7431448254773861395, -0.6691306063588672304, 0.000000000000000000 ) ) ;
#2839=EDGE_LOOP ( 'NONE', ( #1252, #10363, #14918, #2723 ) ) ;
#2850=VECTOR ( 'NONE', #5336, 1000.000000000000000 ) ;
#2855=LINE ( 'NONE', #9172, #10962 ) ;
#2856=ORIENTED_EDGE ( 'NONE', *, *, #11284, .F. ) ;
#2857=ADVANCED_FACE ( 'NONE', ( #9140 ), #236, .F. ) ;
#2865=ADVANCED_FACE ( 'NONE', ( #4401 ), #14826, .T. ) ;
#2869=DIRECTION ( 'NONE',  ( 0.1045284632676436176, 0.9945218953682742891, 0.000000000000000000 ) ) ;
#2876=CARTESIAN_POINT ( 'NONE',  ( 16.34981105473766760, 20.27881147257189909, 102.0000000000000142 ) ) ;
#2880=VERTEX_POINT ( 'NONE', #6665 ) ;
#2881=DIRECTION ( 'NONE',  ( -1.000000000000000000, 0.000000000000000000, 0.000000000000000000 ) ) ;
#2892=AXIS2_PLACEMENT_3D ( 'NONE', #9824, #14875, #2238 ) ;
#2897=ORIENTED_EDGE ( 'NONE', *, *, #3232, .T. ) ;
#2898=DIRECTION ( 'NONE',  ( -0.6691306063588671194, 0.7431448254773861395, 0.000000000000000000 ) ) ;
#2899=ORIENTED_EDGE ( 'NONE', *, *, #2263, .T. ) ;
#2900=ORIENTED_EDGE ( 'NONE', *, *, #9779, .F. ) ;
#2912=EDGE_CURVE ( 'NONE', #12041, #1101, #11793, .T. ) ;
#2926=DIRECTION ( 'NONE',  ( 0.2079116908177531253, 0.9781476007338069101, 0.000000000000000000 ) ) ;
#2929=CARTESIAN_POINT ( 'NONE',  ( 0.000000000000000000, 22.50000000000000000, 101.0000000000000000 ) ) ;
#2942=CARTESIAN_POINT ( 'NONE',  ( -2.464234863135557063, 13.31155363843772932, 101.0000000000000000 ) ) ;
#2947=CARTESIAN_POINT ( 'NONE',  ( -17.45639740057859868, 21.16801284050013976, 101.0000000000000000 ) ) ;
#2957=EDGE_CURVE ( 'NONE', #10320, #10461, #8738, .T. ) ;
#2970=ORIENTED_EDGE ( 'NONE', *, *, #10784, .F. ) ;
#2974=VERTEX_POINT ( 'NONE', #16115 ) ;
#2977=CARTESIAN_POINT ( 'NONE',  ( 0.000000000000000000, 22.50000000000000000, 102.0000000000000142 ) ) ;
#2987=CARTESIAN_POINT ( 'NONE',  ( 16.79120288457601262, 27.43006142852259899, 101.0000000000000000 ) ) ;
#2989=CARTESIAN_POINT ( 'NONE',  ( -1.486087262401750042, 13.10364194761997503, 102.0000000000000142 ) ) ;
#2993=ORIENTED_EDGE ( 'NONE', *, *, #15459, .T. ) ;
#3001=LINE ( 'NONE', #3242, #10790 ) ;
#3002=DIRECTION ( 'NONE',  ( 0.000000000000000000, 0.000000000000000000, 1.000000000000000000 ) ) ;
#3008=CARTESIAN_POINT ( 'NONE',  ( 3.009228475883622522, 5.937825933686468716, 101.6666710451724214 ) ) ;
#3012=DIRECTION ( 'NONE',  ( -0.000000000000000000, -0.000000000000000000, -1.000000000000000000 ) ) ;
#3024=DIRECTION ( 'NONE',  ( 0.9945218953682744001, -0.1045284632676436315, 0.000000000000000000 ) ) ;
#3050=CIRCLE ( 'NONE', #9691, 16.50000000000000711 ) ;
#3052=EDGE_CURVE ( 'NONE', #3406, #793, #8465, .T. ) ;
#3063=CARTESIAN_POINT ( 'NONE',  ( -10.68655108903816142, 8.641875097208238543, 101.0000000000000000 ) ) ;
#3065=DIRECTION ( 'NONE',  ( 0.000000000000000000, 0.000000000000000000, -1.000000000000000000 ) ) ;
#3073=ORIENTED_EDGE ( 'NONE', *, *, #6682, .F. ) ;
#3075=CIRCLE ( 'NONE', #14475, 4.000000000000001776 ) ;
#3080=AXIS2_PLACEMENT_3D ( 'NONE', #6923, #3002, #15795 ) ;
#3083=DIRECTION ( 'NONE',  ( -0.9135454576426005335, -0.4067366430758011520, 0.000000000000000000 ) ) ;
#3085=CARTESIAN_POINT ( 'NONE',  ( 7.394441145214595501, 28.48516834767053751, 102.0000000000000142 ) ) ;
#3098=CONICAL_SURFACE ( 'NONE', #6550, 16.50000000000000711, 0.7853981633974447263 ) ;
#3099=FACE_OUTER_BOUND ( 'NONE', #6152, .T. ) ;
#3103=DIRECTION ( 'NONE',  ( 1.000000000000000000, 0.000000000000000000, -0.000000000000000000 ) ) ;
#3105=AXIS2_PLACEMENT_3D ( 'NONE', #8647, #6413, #4852 ) ;
#3125=EDGE_LOOP ( 'NONE', ( #1944, #433, #2585, #2401, #5991, #9150, #14028, #165, #364, #739, #12218, #8005, #8901, #4818, #16174, #15515, #8971, #325, #10770, #8458, #16106, #12092, #10381, #6476, #14558, #12111, #12135, #5466, #11130, #1660, #11018, #1433, #5804, #1041, #11389, #1636, #7841, #12788, #15811, #3454, #7824, #7645, #10289, #15362, #2377, #14337, #13823, #5145, #11457, #9756, #7319, #2993, #8149, #13317, #5823, #57, #12022, #12258, #13334, #5657, #12176 ) ) ;
#3127=DIRECTION ( 'NONE',  ( -0.9135454576426059736, 0.4067366430757887730, 0.000000000000000000 ) ) ;
#3142=DIRECTION ( 'NONE',  ( -0.8660254037844433705, 0.4999999999999918399, 0.000000000000000000 ) ) ;
#3148=LINE ( 'NONE', #3226, #5441 ) ;
#3152=CARTESIAN_POINT ( 'NONE',  ( -7.436122194756538129, 37.97250723688134855, 101.3333374614808662 ) ) ;
#3156=VERTEX_POINT ( 'NONE', #12779 ) ;
#3169=CARTESIAN_POINT ( 'NONE',  ( 6.000000000000001776, 22.50000000000000000, 101.0000000000000000 ) ) ;
#3197=CARTESIAN_POINT ( 'NONE',  ( -15.83973438765502451, 27.12091057352761325, 102.0000000000000142 ) ) ;
#3199=ORIENTED_EDGE ( 'NONE', *, *, #3603, .F. ) ;
#3207=DIRECTION ( 'NONE',  ( 0.000000000000000000, 0.000000000000000000, -1.000000000000000000 ) ) ;
#3210=B_SPLINE_CURVE_WITH_KNOTS ( 'NONE', 3,
 ( #682, #4117, #7937, #6791 ),
 .UNSPECIFIED., .F., .F.,
 ( 4, 4 ),
 ( 2.829004760666361398E-07, 0.001414802801989365486 ),
 .UNSPECIFIED. ) ;
#3216=ORIENTED_EDGE ( 'NONE', *, *, #15742, .T. ) ;
#3226=CARTESIAN_POINT ( 'NONE',  ( -9.500222237632405253, 22.00424054664139817, 101.0000000000000000 ) ) ;
#3228=LINE ( 'NONE', #2140, #8970 ) ;
#3229=CARTESIAN_POINT ( 'NONE',  ( -6.725310538855818976, 29.22831317314782851, 102.0000000000000142 ) ) ;
#3232=EDGE_CURVE ( 'NONE', #12675, #5661, #1466, .T. ) ;
#3236=ORIENTED_EDGE ( 'NONE', *, *, #6952, .F. ) ;
#3242=CARTESIAN_POINT ( 'NONE',  ( -12.67046914267499069, 34.58135802401869086, 101.0000000000000000 ) ) ;
#3246=LINE ( 'NONE', #9650, #14287 ) ;
#3249=EDGE_CURVE ( 'NONE', #13278, #11303, #15430, .T. ) ;
#3265=B_SPLINE_CURVE_WITH_KNOTS ( 'NONE', 3,
 ( #6465, #15344, #2629, #5070 ),
 .UNSPECIFIED., .F., .F.,
 ( 4, 4 ),
 ( 2.829004760702349710E-07, 0.001414802801989371557 ),
 .UNSPECIFIED. ) ;
#3274=AXIS2_PLACEMENT_3D ( 'NONE', #13919, #3012, #5534 ) ;
#3277=ADVANCED_FACE ( 'NONE', ( #9899 ), #12224, .F. ) ;
#3291=ADVANCED_FACE ( 'NONE', ( #12143 ), #13259, .T. ) ;
#3300=ORIENTED_EDGE ( 'NONE', *, *, #12976, .T. ) ;
#3302=LINE ( 'NONE', #6062, #13938 ) ;
#3313=CARTESIAN_POINT ( 'NONE',  ( 0.000000000000000000, 22.50000000000000000, 102.0000000000000142 ) ) ;
#3320=MANIFOLD_SOLID_BREP ( 'Fillet1', #3352 ) ;
#3328=CARTESIAN_POINT ( 'NONE',  ( 0.000000000000000000, 22.50000000000000000, 101.0000000000000000 ) ) ;
#3329=CARTESIAN_POINT ( 'NONE',  ( -3.407225380398804404, 31.38205016914259105, 101.0000000000000000 ) ) ;
#3340=CARTESIAN_POINT ( 'NONE',  ( 1.486087262401875941, 13.10364194761998213, 101.0000000000000000 ) ) ;
#3342=VECTOR ( 'NONE', #474, 1000.000000000000000 ) ;
#3344=LINE ( 'NONE', #3435, #5713 ) ;
#3352=CLOSED_SHELL ( 'NONE', ( #340, #9425, #15061, #4596, #4600, #11997, #15540, #5614, #13028, #2865, #5348, #4130, #1831, #11349, #7416, #15151, #9005, #1139, #10596, #10379, #6482, #5246, #11840, #1524, #11929, #9065, #5107, #13308, #4482, #13095, #9438, #11226, #5373, #2857, #2046, #13588, #6077, #518, #7037, #12212, #1037, #7763, #1376, #7530, #142, #6647, #6327, #1109, #7467, #3681, #7130, #9163, #5608, #12112, #14525, #10180, #12714, #14320, #14720, #6203, #2698, #2301, #12507, #12901, #1662, #1859, #15961, #4443, #10602, #10069, #13449, #4386, #7968, #3277, #1033, #7787, #1115, #6416, #4197, #10285, #2557, #9876, #11225, #5615, #12804, #3291 ) ) ;
#3355=AXIS2_PLACEMENT_3D ( 'NONE', #10740, #1991, #4768 ) ;
#3356=AXIS2_PLACEMENT_3D ( 'NONE', #8664, #9761, #845 ) ;
#3362=EDGE_CURVE ( 'NONE', #566, #4055, #833, .T. ) ;
#3368=EDGE_LOOP ( 'NONE', ( #3979, #7984, #15935, #2640 ) ) ;
#3369=VECTOR ( 'NONE', #13704, 1000.000000000000000 ) ;
#3388=ORIENTED_EDGE ( 'NONE', *, *, #1841, .T. ) ;
#3390=VECTOR ( 'NONE', #13536, 999.9999999999998863 ) ;
#3396=PLANE ( 'NONE',  #12957 ) ;
#3402=CARTESIAN_POINT ( 'NONE',  ( 0.000000000000000000, 22.50000000000000000, 101.0000000000000000 ) ) ;
#3405=CARTESIAN_POINT ( 'NONE',  ( -5.988468393965924008, 15.10823117958422301, 101.0000000000000000 ) ) ;
#3406=VERTEX_POINT ( 'NONE', #4926 ) ;
#3409=ORIENTED_EDGE ( 'NONE', *, *, #2651, .T. ) ;
#3414=CARTESIAN_POINT ( 'NONE',  ( 16.34981105473766760, 20.27881147257189909, 102.0000000000000142 ) ) ;
#3415=ORIENTED_EDGE ( 'NONE', *, *, #15135, .F. ) ;
#3426=( NAMED_UNIT ( * ) SI_UNIT ( $, .STERADIAN. ) SOLID_ANGLE_UNIT ( ) );
#3435=CARTESIAN_POINT ( 'NONE',  ( 5.179451399591075145, 14.52044592729181538, 101.0000000000000000 ) ) ;
#3439=DIRECTION ( 'NONE',  ( -0.000000000000000000, 0.000000000000000000, 1.000000000000000000 ) ) ;
#3451=ORIENTED_EDGE ( 'NONE', *, *, #5460, .F. ) ;
#3454=ORIENTED_EDGE ( 'NONE', *, *, #11284, .T. ) ;
#3464=EDGE_CURVE ( 'NONE', #9110, #1819, #13528, .T. ) ;
#3468=EDGE_LOOP ( 'NONE', ( #3472, #15630, #4022, #16418 ) ) ;
#3472=ORIENTED_EDGE ( 'NONE', *, *, #7941, .F. ) ;
#3474=ORIENTED_EDGE ( 'NONE', *, *, #5567, .T. ) ;
#3476=CARTESIAN_POINT ( 'NONE',  ( 17.50000000000000000, 22.50000000000000355, 80.00000000000000000 ) ) ;
#3477=EDGE_CURVE ( 'NONE', #8881, #9739, #3909, .T. ) ;
#3488=EDGE_LOOP ( 'NONE', ( #13018, #12960, #9890, #4639 ) ) ;
#3489=EDGE_CURVE ( 'NONE', #15672, #5969, #2323, .T. ) ;
#3491=ORIENTED_EDGE ( 'NONE', *, *, #2957, .T. ) ;
#3493=ORIENTED_EDGE ( 'NONE', *, *, #9782, .T. ) ;
#3500=FILL_AREA_STYLE_COLOUR ( '', #9281 ) ;
#3505=DIRECTION ( 'NONE',  ( 0.000000000000000000, 0.000000000000000000, -1.000000000000000000 ) ) ;
#3506=DIRECTION ( 'NONE',  ( 0.000000000000000000, -0.000000000000000000, 1.000000000000000000 ) ) ;
#3507=PLANE ( 'NONE',  #8590 ) ;
#3513=DIRECTION ( 'NONE',  ( 0.000000000000000000, 0.000000000000000000, 1.000000000000000000 ) ) ;
#3517=EDGE_LOOP ( 'NONE', ( #14869, #5824, #12490, #11784 ) ) ;
#3518=DIRECTION ( 'NONE',  ( 0.8660254037844362651, 0.5000000000000041078, 0.000000000000000000 ) ) ;
#3523=DIRECTION ( 'NONE',  ( 0.000000000000000000, 0.000000000000000000, -1.000000000000000000 ) ) ;
#3535=EDGE_CURVE ( 'NONE', #14691, #14151, #5850, .T. ) ;
#3556=DIRECTION ( 'NONE',  ( 0.5000000000000041078, -0.8660254037844363761, -0.000000000000000000 ) ) ;
#3557=CARTESIAN_POINT ( 'NONE',  ( -16.79120288457607657, 27.43006142852237517, 101.0000000000000000 ) ) ;
#3563=VECTOR ( 'NONE', #12126, 999.9999999999998863 ) ;
#3565=CARTESIAN_POINT ( 'NONE',  ( 13.33959974903368995, 33.83821319854147447, 101.0000000000000000 ) ) ;
#3572=ORIENTED_EDGE ( 'NONE', *, *, #2125, .F. ) ;
#3578=ORIENTED_EDGE ( 'NONE', *, *, #2254, .F. ) ;
#3585=EDGE_CURVE ( 'NONE', #5800, #7317, #15393, .T. ) ;
#3590=CIRCLE ( 'NONE', #8089, 17.50000000000000000 ) ;
#3597=ORIENTED_EDGE ( 'NONE', *, *, #1100, .F. ) ;
#3603=EDGE_CURVE ( 'NONE', #4080, #9526, #1047, .T. ) ;
#3612=PLANE ( 'NONE',  #11861 ) ;
#3620=VECTOR ( 'NONE', #1929, 1000.000000000000114 ) ;
#3639=CIRCLE ( 'NONE', #15298, 17.50000000000000000 ) ;
#3640=VECTOR ( 'NONE', #12630, 1000.000000000000000 ) ;
#3647=CARTESIAN_POINT ( 'NONE',  ( 17.11764542475610185, 21.20361710786393417, 101.3333374614808662 ) ) ;
#3654=PLANE ( 'NONE',  #8592 ) ;
#3657=EDGE_LOOP ( 'NONE', ( #5872, #13522, #6637, #8547 ) ) ;
#3667=DIRECTION ( 'NONE',  ( -0.000000000000000000, 0.000000000000000000, 1.000000000000000000 ) ) ;
#3669=CARTESIAN_POINT ( 'NONE',  ( 0.000000000000000000, 22.50000000000000000, 102.0000000000000142 ) ) ;
#3673=LINE ( 'NONE', #8729, #4421 ) ;
#3674=AXIS2_PLACEMENT_3D ( 'NONE', #6394, #6226, #3897 ) ;
#3681=ADVANCED_FACE ( 'NONE', ( #6486 ), #144, .F. ) ;
#3688=CARTESIAN_POINT ( 'NONE',  ( -17.45639740057859868, 21.16801284050013976, 102.0000000000000142 ) ) ;
#3690=DIRECTION ( 'NONE',  ( 0.000000000000000000, 0.000000000000000000, -1.000000000000000000 ) ) ;
#3691=CARTESIAN_POINT ( 'NONE',  ( 0.000000000000000000, 22.50000000000000000, 102.0000000000000142 ) ) ;
#3706=ORIENTED_EDGE ( 'NONE', *, *, #12556, .T. ) ;
#3716=AXIS2_PLACEMENT_3D ( 'NONE', #2572, #6405, #7726 ) ;
#3721=ORIENTED_EDGE ( 'NONE', *, *, #11682, .F. ) ;
#3726=DIRECTION ( 'NONE',  ( 0.8090169943749425663, 0.5877852522924799095, 0.000000000000000000 ) ) ;
#3739=CARTESIAN_POINT ( 'NONE',  ( -7.977241335952133916, 17.31698729810774751, 102.0000000000000142 ) ) ;
#3740=DIRECTION ( 'NONE',  ( -1.000000000000000000, 0.000000000000000000, 0.000000000000000000 ) ) ;
#3744=DIRECTION ( 'NONE',  ( 0.000000000000000000, 0.000000000000000000, 1.000000000000000000 ) ) ;
#3746=PLANE ( 'NONE',  #15092 ) ;
#3747=CARTESIAN_POINT ( 'NONE',  ( 0.5000000000000001110, 38.99242250247064590, 102.0000000000000142 ) ) ;
#3755=CARTESIAN_POINT ( 'NONE',  ( -10.68655108903816142, 8.641875097208238543, 101.0000000000000000 ) ) ;
#3771=DIRECTION ( 'NONE',  ( 0.000000000000000000, 0.000000000000000000, 1.000000000000000000 ) ) ;
#3782=ORIENTED_EDGE ( 'NONE', *, *, #2358, .T. ) ;
#3785=DIRECTION ( 'NONE',  ( -0.2079116908177665313, 0.9781476007338041345, 0.000000000000000000 ) ) ;
#3787=CARTESIAN_POINT ( 'NONE',  ( -2.939893647802529930, 6.264020653511205516, 102.0000000000000142 ) ) ;
#3810=CARTESIAN_POINT ( 'NONE',  ( 0.000000000000000000, 22.50000000000000000, 102.0000000000000142 ) ) ;
#3818=EDGE_LOOP ( 'NONE', ( #11485, #6594 ) ) ;
#3819=VERTEX_POINT ( 'NONE', #13360 ) ;
#3820=EDGE_CURVE ( 'NONE', #7211, #9602, #6812, .T. ) ;
#3822=DIRECTION ( 'NONE',  ( 0.000000000000000000, 0.000000000000000000, 1.000000000000000000 ) ) ;
#3823=VECTOR ( 'NONE', #5344, 1000.000000000000000 ) ;
#3827=DIRECTION ( 'NONE',  ( -0.2079116908177665590, 0.9781476007338041345, 0.000000000000000000 ) ) ;
#3844=FACE_OUTER_BOUND ( 'NONE', #1249, .T. ) ;
#3852=DIRECTION ( 'NONE',  ( 1.000000000000000000, 1.784287003861858816E-14, 0.000000000000000000 ) ) ;
#3857=ORIENTED_EDGE ( 'NONE', *, *, #7088, .T. ) ;
#3858=VERTEX_POINT ( 'NONE', #724 ) ;
#3861=ORIENTED_EDGE ( 'NONE', *, *, #5945, .T. ) ;
#3867=DIRECTION ( 'NONE',  ( -1.000000000000000000, 0.000000000000000000, 0.000000000000000000 ) ) ;
#3871=EDGE_CURVE ( 'NONE', #9378, #15183, #7852, .T. ) ;
#3877=EDGE_CURVE ( 'NONE', #14668, #14510, #6823, .T. ) ;
#3879=ORIENTED_EDGE ( 'NONE', *, *, #10122, .F. ) ;
#3880=CIRCLE ( 'NONE', #11851, 17.50000000000000000 ) ;
#3881=VECTOR ( 'NONE', #6264, 1000.000000000000000 ) ;
#3884=DIRECTION ( 'NONE',  ( -0.9510565162951544194, 0.3090169943749449533, 0.000000000000000000 ) ) ;
#3885=DIRECTION ( 'NONE',  ( 0.000000000000000000, 0.000000000000000000, 1.000000000000000000 ) ) ;
#3893=CIRCLE ( 'NONE', #10789, 2.000000000000001776 ) ;
#3895=DIRECTION ( 'NONE',  ( 0.4067366430757888285, 0.9135454576426059736, 0.000000000000000000 ) ) ;
#3897=DIRECTION ( 'NONE',  ( 0.5000000000000039968, -0.8660254037844363761, 0.000000000000000000 ) ) ;
#3898=CARTESIAN_POINT ( 'NONE',  ( 6.661118525004998681, 38.69041383028350367, 101.0000000000000000 ) ) ;
#3901=VERTEX_POINT ( 'NONE', #12116 ) ;
#3909=LINE ( 'NONE', #10142, #10092 ) ;
#3911=LINE ( 'NONE', #2654, #15023 ) ;
#3917=AXIS2_PLACEMENT_3D ( 'NONE', #1404, #2492, #2580 ) ;
#3935=CARTESIAN_POINT ( 'NONE',  ( -17.50000000000000000, 22.50000000000000000, 80.00000000000000000 ) ) ;
#3960=EDGE_CURVE ( 'NONE', #7907, #14575, #4485, .T. ) ;
#3971=AXIS2_PLACEMENT_3D ( 'NONE', #15884, #7241, #4507 ) ;
#3977=ORIENTED_EDGE ( 'NONE', *, *, #10152, .T. ) ;
#3979=ORIENTED_EDGE ( 'NONE', *, *, #281, .T. ) ;
#3985=CARTESIAN_POINT ( 'NONE',  ( -7.394441145214675437, 28.48516834767043093, 101.0000000000000000 ) ) ;
#3986=CARTESIAN_POINT ( 'NONE',  ( 0.000000000000000000, 22.50000000000000000, 102.0000000000000142 ) ) ;
#3994=CARTESIAN_POINT ( 'NONE',  ( 16.48898053797764973, 28.38332565970932819, 101.0000000000000000 ) ) ;
#3996=CARTESIAN_POINT ( 'NONE',  ( 13.33959974903368995, 33.83821319854147447, 102.0000000000000142 ) ) ;
#4007=ORIENTED_EDGE ( 'NONE', *, *, #10918, .T. ) ;
#4022=ORIENTED_EDGE ( 'NONE', *, *, #711, .F. ) ;
#4040=CARTESIAN_POINT ( 'NONE',  ( -5.179451399590974781, 14.52044592729175321, 102.0000000000000142 ) ) ;
#4041=EDGE_LOOP ( 'NONE', ( #10343, #14539, #2970, #8925, #7296 ) ) ;
#4046=LINE ( 'NONE', #13847, #14738 ) ;
#4049=CARTESIAN_POINT ( 'NONE',  ( 0.5000000000000000000, 39.65938208326293335, 101.3333374618097480 ) ) ;
#4050=CARTESIAN_POINT ( 'NONE',  ( -0.5000000000000000000, 39.99999999999999289, 101.0000000000000000 ) ) ;
#4054=CARTESIAN_POINT ( 'NONE',  ( -5.988468393965924008, 15.10823117958422301, 101.0000000000000000 ) ) ;
#4055=VERTEX_POINT ( 'NONE', #8533 ) ;
#4058=ORIENTED_EDGE ( 'NONE', *, *, #13590, .T. ) ;
#4064=DIRECTION ( 'NONE',  ( -0.6691306063588567943, -0.7431448254773955764, 0.000000000000000000 ) ) ;
#4076=CARTESIAN_POINT ( 'NONE',  ( -6.386939227490606719, 38.07459704542236523, 101.6666710451724214 ) ) ;
#4080=VERTEX_POINT ( 'NONE', #10125 ) ;
#4081=EDGE_CURVE ( 'NONE', #16202, #4152, #4046, .T. ) ;
#4090=DIRECTION ( 'NONE',  ( -0.6691306063588671194, 0.7431448254773862505, 0.000000000000000000 ) ) ;
#4107=EDGE_CURVE ( 'NONE', #8153, #12133, #8957, .T. ) ;
#4117=CARTESIAN_POINT ( 'NONE',  ( -9.681523229999493552, 8.323875655254827421, 101.3333374614808662 ) ) ;
#4124=ORIENTED_EDGE ( 'NONE', *, *, #4192, .F. ) ;
#4126=EDGE_LOOP ( 'NONE', ( #9510, #4963, #2897, #13373 ) ) ;
#4128=DIRECTION ( 'NONE',  ( 0.000000000000000000, -0.000000000000000000, 1.000000000000000000 ) ) ;
#4129=AXIS2_PLACEMENT_3D ( 'NONE', #8131, #5337, #9306 ) ;
#4130=ADVANCED_FACE ( 'NONE', ( #14012 ), #4687, .T. ) ;
#4135=COLOUR_RGB ( '', 0.31764706, 0.68627451, 0.89019608) ;
#4142=DIRECTION ( 'NONE',  ( -0.4067366430757887175, -0.9135454576426059736, 0.000000000000000000 ) ) ;
#4144=VECTOR ( 'NONE', #1393, 1000.000000000000000 ) ;
#4146=AXIS2_PLACEMENT_3D ( 'NONE', #3669, #8726, #11157 ) ;
#4151=EDGE_LOOP ( 'NONE', ( #12411, #16082, #9528, #12192 ) ) ;
#4152=VERTEX_POINT ( 'NONE', #12697 ) ;
#4159=AXIS2_PLACEMENT_3D ( 'NONE', #12148, #4587, #4429 ) ;
#4160=VECTOR ( 'NONE', #6022, 999.9999999999998863 ) ;
#4168=DIRECTION ( 'NONE',  ( 1.000000000000000000, 0.000000000000000000, 0.000000000000000000 ) ) ;
#4174=AXIS2_PLACEMENT_3D ( 'NONE', #11695, #1151, #11160 ) ;
#4178=DIRECTION ( 'NONE',  ( 1.224646799147353207E-16, -1.000000000000000000, 0.000000000000000000 ) ) ;
#4184=DIRECTION ( 'NONE',  ( 0.000000000000000000, 0.000000000000000000, -1.000000000000000000 ) ) ;
#4192=EDGE_CURVE ( 'NONE', #15550, #14671, #8195, .T. ) ;
#4197=ADVANCED_FACE ( 'NONE', ( #14093 ), #4987, .F. ) ;
#4215=ORIENTED_EDGE ( 'NONE', *, *, #15916, .T. ) ;
#4242=MECHANICAL_DESIGN_GEOMETRIC_PRESENTATION_REPRESENTATION('',(#2096),#15381);
#4253=EDGE_LOOP ( 'NONE', ( #4261, #3597, #8546, #5666 ) ) ;
#4261=ORIENTED_EDGE ( 'NONE', *, *, #307, .F. ) ;
#4274=CARTESIAN_POINT ( 'NONE',  ( 13.33429048796497085, 33.83343271840296751, 101.0000000000000000 ) ) ;
#4275=VERTEX_POINT ( 'NONE', #4379 ) ;
#4278=EDGE_CURVE ( 'NONE', #9110, #7461, #10377, .T. ) ;
#4287=LINE ( 'NONE', #5619, #3620 ) ;
#4292=EDGE_CURVE ( 'NONE', #6085, #10405, #7038, .T. ) ;
#4313=ORIENTED_EDGE ( 'NONE', *, *, #1100, .T. ) ;
#4327=VECTOR ( 'NONE', #13055, 999.9999999999998863 ) ;
#4332=VERTEX_POINT ( 'NONE', #4626 ) ;
#4337=DIRECTION ( 'NONE',  ( 0.000000000000000000, 0.000000000000000000, -1.000000000000000000 ) ) ;
#4350=CARTESIAN_POINT ( 'NONE',  ( 2.939893647802748866, 6.264020653511243708, 102.0000000000000142 ) ) ;
#4373=ORIENTED_EDGE ( 'NONE', *, *, #16278, .F. ) ;
#4379=CARTESIAN_POINT ( 'NONE',  ( -8.880528407616480990, 25.91118970470954963, 102.0000000000000142 ) ) ;
#4382=PLANE ( 'NONE',  #385 ) ;
#4386=ADVANCED_FACE ( 'NONE', ( #13423 ), #15923, .T. ) ;
#4389=ORIENTED_EDGE ( 'NONE', *, *, #4643, .T. ) ;
#4394=CIRCLE ( 'NONE', #13670, 17.50000000000000000 ) ;
#4401=FACE_OUTER_BOUND ( 'NONE', #16328, .T. ) ;
#4404=CARTESIAN_POINT ( 'NONE',  ( 8.880528407616436581, 25.91118970470966687, 101.0000000000000000 ) ) ;
#4407=DIRECTION ( 'NONE',  ( -0.8660254037844363761, -0.5000000000000039968, 0.000000000000000000 ) ) ;
#4408=DIRECTION ( 'NONE',  ( -0.3090169943749448977, -0.9510565162951543083, 0.000000000000000000 ) ) ;
#4412=ORIENTED_EDGE ( 'NONE', *, *, #13630, .F. ) ;
#4421=VECTOR ( 'NONE', #7485, 999.9999999999998863 ) ;
#4427=CARTESIAN_POINT ( 'NONE',  ( 9.881733417930924190, 8.048309972292271297, 102.0000000000000142 ) ) ;
#4429=DIRECTION ( 'NONE',  ( 1.000000000000000000, 7.930164461608261426E-16, 0.000000000000000000 ) ) ;
#4433=DIRECTION ( 'NONE',  ( -0.2079116908177665313, 0.9781476007338041345, 0.000000000000000000 ) ) ;
#4438=VECTOR ( 'NONE', #14211, 1000.000000000000000 ) ;
#4441=UNCERTAINTY_MEASURE_WITH_UNIT (LENGTH_MEASURE( 1.000000000000000082E-05 ), #7325, 'distance_accuracy_value', 'NONE');
#4443=ADVANCED_FACE ( 'NONE', ( #8440 ), #7198, .T. ) ;
#4460=EDGE_LOOP ( 'NONE', ( #1584, #16260, #2, #8764 ) ) ;
#4470=CARTESIAN_POINT ( 'NONE',  ( 0.000000000000000000, 22.50000000000000000, 102.0000000000000142 ) ) ;
#4479=ORIENTED_EDGE ( 'NONE', *, *, #399, .T. ) ;
#4482=ADVANCED_FACE ( 'NONE', ( #10189 ), #9023, .T. ) ;
#4484=CARTESIAN_POINT ( 'NONE',  ( 15.40544456622774661, 14.18301270189236973, 101.0000000000000000 ) ) ;
#4485=LINE ( 'NONE', #16349, #13418 ) ;
#4495=DIRECTION ( 'NONE',  ( 0.000000000000000000, 0.000000000000000000, 1.000000000000000000 ) ) ;
#4499=VERTEX_POINT ( 'NONE', #6371 ) ;
#4507=DIRECTION ( 'NONE',  ( 1.000000000000000000, 0.000000000000000000, 0.000000000000000000 ) ) ;
#4515=DIRECTION ( 'NONE',  ( 0.000000000000000000, 0.000000000000000000, -1.000000000000000000 ) ) ;
#4517=CARTESIAN_POINT ( 'NONE',  ( 7.571758127758665857, 38.27715053026751946, 101.0000000000000000 ) ) ;
#4521=B_SPLINE_CURVE_WITH_KNOTS ( 'NONE', 3,
 ( #8639, #989, #2236, #2325 ),
 .UNSPECIFIED., .F., .F.,
 ( 4, 4 ),
 ( 2.829004760679149478E-07, 0.001414802801989367221 ),
 .UNSPECIFIED. ) ;
#4545=DIRECTION ( 'NONE',  ( 0.9781476007338070211, -0.2079116908177531808, -0.000000000000000000 ) ) ;
#4548=FACE_OUTER_BOUND ( 'NONE', #1563, .T. ) ;
#4554=ORIENTED_EDGE ( 'NONE', *, *, #794, .F. ) ;
#4557=ORIENTED_EDGE ( 'NONE', *, *, #4278, .T. ) ;
#4567=CARTESIAN_POINT ( 'NONE',  ( 0.000000000000000000, 22.50000000000000000, 101.0000000000000000 ) ) ;
#4587=DIRECTION ( 'NONE',  ( 0.000000000000000000, 0.000000000000000000, -1.000000000000000000 ) ) ;
#4596=ADVANCED_FACE ( 'NONE', ( #16423 ), #8377, .T. ) ;
#4600=ADVANCED_FACE ( 'NONE', ( #4972 ), #8937, .T. ) ;
#4601=UNCERTAINTY_MEASURE_WITH_UNIT (LENGTH_MEASURE( 1.000000000000000082E-05 ), #8405, 'distance_accuracy_value', 'NONE');
#4602=CARTESIAN_POINT ( 'NONE',  ( 16.45433951800531247, 21.27333336794017171, 102.0000000000000142 ) ) ;
#4613=FACE_OUTER_BOUND ( 'NONE', #6526, .T. ) ;
#4622=EDGE_CURVE ( 'NONE', #11153, #5800, #12168, .T. ) ;
#4624=CIRCLE ( 'NONE', #10973, 16.50000000000000711 ) ;
#4626=CARTESIAN_POINT ( 'NONE',  ( 10.68655108903834794, 8.641875097208380652, 101.0000000000000000 ) ) ;
#4636=ORIENTED_EDGE ( 'NONE', *, *, #7662, .F. ) ;
#4639=ORIENTED_EDGE ( 'NONE', *, *, #5117, .F. ) ;
#4643=EDGE_CURVE ( 'NONE', #9526, #4080, #16099, .T. ) ;
#4644=LINE ( 'NONE', #5889, #15591 ) ;
#4645=CARTESIAN_POINT ( 'NONE',  ( 16.48218589020105185, 28.38111794481774908, 101.0000000000000000 ) ) ;
#4656=CARTESIAN_POINT ( 'NONE',  ( 17.34476375915451740, 20.17423772944865945, 101.0000000000000000 ) ) ;
#4661=ORIENTED_EDGE ( 'NONE', *, *, #13801, .T. ) ;
#4674=DIRECTION ( 'NONE',  ( 1.000000000000000000, 0.000000000000000000, 0.000000000000000000 ) ) ;
#4680=PLANE ( 'NONE',  #6048 ) ;
#4681=B_SPLINE_CURVE_WITH_KNOTS ( 'NONE', 3,
 ( #2063, #3152, #5586, #7065 ),
 .UNSPECIFIED., .F., .F.,
 ( 4, 4 ),
 ( 2.829004760709176796E-07, 0.001414802801989367871 ),
 .UNSPECIFIED. ) ;
#4685=DIRECTION ( 'NONE',  ( 0.000000000000000000, 0.000000000000000000, -1.000000000000000000 ) ) ;
#4687=CONICAL_SURFACE ( 'NONE', #150, 16.50000000000000711, 0.7853981633974447263 ) ;
#4717=CIRCLE ( 'NONE', #16368, 17.50000000000000000 ) ;
#4718=AXIS2_PLACEMENT_3D ( 'NONE', #6244, #14179, #6164 ) ;
#4719=VECTOR ( 'NONE', #2837, 1000.000000000000000 ) ;
#4730=AXIS2_PLACEMENT_3D ( 'NONE', #7216, #3556, #878 ) ;
#4741=DIRECTION ( 'NONE',  ( -0.000000000000000000, -0.000000000000000000, -1.000000000000000000 ) ) ;
#4751=EDGE_CURVE ( 'NONE', #3156, #7423, #1762, .T. ) ;
#4761=ORIENTED_EDGE ( 'NONE', *, *, #4751, .F. ) ;
#4767=PLANE ( 'NONE',  #2892 ) ;
#4768=DIRECTION ( 'NONE',  ( -1.000000000000000000, 0.000000000000000000, 0.000000000000000000 ) ) ;
#4776=CARTESIAN_POINT ( 'NONE',  ( 0.000000000000000000, 22.50000000000000000, 101.0000000000000000 ) ) ;
#4780=DIRECTION ( 'NONE',  ( 0.9945218953682730678, 0.1045284632676572317, 0.000000000000000000 ) ) ;
#4782=EDGE_CURVE ( 'NONE', #4820, #14671, #6827, .T. ) ;
#4783=CARTESIAN_POINT ( 'NONE',  ( 14.32166083077716578, 13.65403499491884354, 101.6666710451724214 ) ) ;
#4784=LINE ( 'NONE', #11092, #10775 ) ;
#4788=VECTOR ( 'NONE', #6561, 1000.000000000000000 ) ;
#4791=CARTESIAN_POINT ( 'NONE',  ( 6.661118525004998681, 38.69041383028350367, 101.0000000000000000 ) ) ;
#4798=B_SPLINE_CURVE_WITH_KNOTS ( 'NONE', 3,
 ( #3063, #9235, #15697, #9143 ),
 .UNSPECIFIED., .F., .F.,
 ( 4, 4 ),
 ( 2.829004760700636057E-07, 0.001414802801989368088 ),
 .UNSPECIFIED. ) ;
#4818=ORIENTED_EDGE ( 'NONE', *, *, #13824, .T. ) ;
#4820=VERTEX_POINT ( 'NONE', #6025 ) ;
#4827=CARTESIAN_POINT ( 'NONE',  ( 0.000000000000000000, 22.50000000000000000, 102.0000000000000142 ) ) ;
#4833=EDGE_LOOP ( 'NONE', ( #5425, #13001, #1897, #4124 ) ) ;
#4841=VERTEX_POINT ( 'NONE', #10920 ) ;
#4844=DIRECTION ( 'NONE',  ( 0.2079116908177531531, 0.9781476007338069101, 0.000000000000000000 ) ) ;
#4845=FACE_OUTER_BOUND ( 'NONE', #10162, .T. ) ;
#4852=DIRECTION ( 'NONE',  ( -1.000000000000000000, 0.000000000000000000, 0.000000000000000000 ) ) ;
#4865=CARTESIAN_POINT ( 'NONE',  ( -15.40544456622763470, 14.18301270189214947, 102.0000000000000142 ) ) ;
#4866=CARTESIAN_POINT ( 'NONE',  ( -6.658212670116278709, 38.68388717334321569, 101.0000000000000000 ) ) ;
#4886=DIRECTION ( 'NONE',  ( 0.9781476007338042455, 0.2079116908177664758, 0.000000000000000000 ) ) ;
#4900=FACE_OUTER_BOUND ( 'NONE', #12337, .T. ) ;
#4907=EDGE_CURVE ( 'NONE', #8817, #7744, #12742, .T. ) ;
#4914=ORIENTED_EDGE ( 'NONE', *, *, #7088, .F. ) ;
#4916=ORIENTED_EDGE ( 'NONE', *, *, #12556, .F. ) ;
#4919=AXIS2_PLACEMENT_3D ( 'NONE', #2942, #11751, #10348 ) ;
#4924=ORIENTED_EDGE ( 'NONE', *, *, #9988, .T. ) ;
#4926=CARTESIAN_POINT ( 'NONE',  ( -3.407225380398804404, 31.38205016914259105, 101.0000000000000000 ) ) ;
#4928=PLANE ( 'NONE',  #12639 ) ;
#4941=EDGE_LOOP ( 'NONE', ( #1372, #1547, #549, #12772 ) ) ;
#4946=AXIS2_PLACEMENT_3D ( 'NONE', #14762, #4741, #8532 ) ;
#4947=CARTESIAN_POINT ( 'NONE',  ( 16.48218589020105185, 28.38111794481774908, 101.0000000000000000 ) ) ;
#4948=LINE ( 'NONE', #13264, #3881 ) ;
#4963=ORIENTED_EDGE ( 'NONE', *, *, #10194, .F. ) ;
#4968=PLANE ( 'NONE',  #2505 ) ;
#4969=CIRCLE ( 'NONE', #13182, 16.50000000000000711 ) ;
#4971=VECTOR ( 'NONE', #7808, 1000.000000000000000 ) ;
#4972=FACE_OUTER_BOUND ( 'NONE', #1040, .T. ) ;
#4987=PLANE ( 'NONE',  #14210 ) ;
#4990=EDGE_CURVE ( 'NONE', #1326, #895, #1262, .T. ) ;
#4996=DIRECTION ( 'NONE',  ( -0.9135454576426059736, 0.4067366430757888285, 0.000000000000000000 ) ) ;
#5008=FACE_OUTER_BOUND ( 'NONE', #7985, .T. ) ;
#5017=DIRECTION ( 'NONE',  ( -0.000000000000000000, 0.000000000000000000, 1.000000000000000000 ) ) ;
#5026=ORIENTED_EDGE ( 'NONE', *, *, #5316, .F. ) ;
#5031=DIRECTION ( 'NONE',  ( 0.000000000000000000, 0.000000000000000000, 1.000000000000000000 ) ) ;
#5043=CIRCLE ( 'NONE', #12460, 16.50000000000000711 ) ;
#5048=B_SPLINE_CURVE_WITH_KNOTS ( 'NONE', 3,
 ( #14963, #15126, #7489, #2411 ),
 .UNSPECIFIED., .F., .F.,
 ( 4, 4 ),
 ( 2.829004760659353259E-07, 0.001414802801989363968 ),
 .UNSPECIFIED. ) ;
#5052=ORIENTED_EDGE ( 'NONE', *, *, #11589, .T. ) ;
#5067=CARTESIAN_POINT ( 'NONE',  ( 17.01311696148846053, 20.20909521249566154, 101.3333374614808662 ) ) ;
#5070=CARTESIAN_POINT ( 'NONE',  ( -11.92169313911859341, 33.90715708214334256, 102.0000000000000142 ) ) ;
#5077=FACE_OUTER_BOUND ( 'NONE', #4041, .T. ) ;
#5078=DIRECTION ( 'NONE',  ( -1.000000000000000000, 0.000000000000000000, 0.000000000000000000 ) ) ;
#5104=ORIENTED_EDGE ( 'NONE', *, *, #4278, .F. ) ;
#5107=ADVANCED_FACE ( 'NONE', ( #8164 ), #10586, .F. ) ;
#5109=LINE ( 'NONE', #1336, #14479 ) ;
#5117=EDGE_CURVE ( 'NONE', #7989, #10461, #3893, .T. ) ;
#5129=ORIENTED_EDGE ( 'NONE', *, *, #6117, .F. ) ;
#5130=ORIENTED_EDGE ( 'NONE', *, *, #11795, .F. ) ;
#5133=FACE_OUTER_BOUND ( 'NONE', #9934, .T. ) ;
#5142=CARTESIAN_POINT ( 'NONE',  ( 17.34476375915451740, 20.17423772944865945, 101.0000000000000000 ) ) ;
#5143=ORIENTED_EDGE ( 'NONE', *, *, #4081, .F. ) ;
#5145=ORIENTED_EDGE ( 'NONE', *, *, #3249, .T. ) ;
#5147=LINE ( 'NONE', #6466, #16335 ) ;
#5153=FACE_OUTER_BOUND ( 'NONE', #6481, .T. ) ;
#5154=AXIS2_PLACEMENT_3D ( 'NONE', #2929, #7996, #338 ) ;
#5159=EDGE_CURVE ( 'NONE', #14171, #7383, #6605, .T. ) ;
#5160=ORIENTED_EDGE ( 'NONE', *, *, #3960, .F. ) ;
#5166=CONICAL_SURFACE ( 'NONE', #5688, 16.50000000000000711, 0.7853981633974447263 ) ;
#5167=DIRECTION ( 'NONE',  ( 0.000000000000000000, 0.000000000000000000, 1.000000000000000000 ) ) ;
#5170=LINE ( 'NONE', #10144, #16356 ) ;
#5179=ORIENTED_EDGE ( 'NONE', *, *, #283, .T. ) ;
#5180=VECTOR ( 'NONE', #13031, 1000.000000000000000 ) ;
#5186=ORIENTED_EDGE ( 'NONE', *, *, #9680, .F. ) ;
#5189=VECTOR ( 'NONE', #8202, 1000.000000000000000 ) ;
#5200=EDGE_CURVE ( 'NONE', #11991, #14378, #4969, .T. ) ;
#5203=AXIS2_PLACEMENT_3D ( 'NONE', #7541, #3885, #15255 ) ;
#5206=ORIENTED_EDGE ( 'NONE', *, *, #8853, .F. ) ;
#5220=PRODUCT ( 'Speed Control Knob & Dial', 'Speed Control Knob & Dial', '', ( #13346 ) ) ;
#5230=AXIS2_PLACEMENT_3D ( 'NONE', #5469, #15598, #9286 ) ;
#5231=AXIS2_PLACEMENT_3D ( 'NONE', #3328, #2076, #828 ) ;
#5243=AXIS2_PLACEMENT_3D ( 'NONE', #12325, #3523, #9844 ) ;
#5246=ADVANCED_FACE ( 'NONE', ( #13629 ), #2819, .T. ) ;
#5252=CARTESIAN_POINT ( 'NONE',  ( 7.394441145214595501, 28.48516834767053751, 101.0000000000000000 ) ) ;
#5254=ORIENTED_EDGE ( 'NONE', *, *, #13416, .F. ) ;
#5255=CIRCLE ( 'NONE', #11607, 17.50000000000000000 ) ;
#5256=EDGE_CURVE ( 'NONE', #7399, #4332, #11327, .T. ) ;
#5257=CARTESIAN_POINT ( 'NONE',  ( 0.000000000000000000, 22.50000000000000000, 102.0000000000000142 ) ) ;
#5258=CARTESIAN_POINT ( 'NONE',  ( -9.877534094663211306, 8.054089844915763408, 101.0000000000000000 ) ) ;
#5259=DIRECTION ( 'NONE',  ( 0.000000000000000000, 0.000000000000000000, -1.000000000000000000 ) ) ;
#5260=CARTESIAN_POINT ( 'NONE',  ( 12.67046914267482016, 34.58135802401886139, 102.0000000000000142 ) ) ;
#5261=DIRECTION ( 'NONE',  ( -0.9945218953682744001, 0.1045284632676435066, 0.000000000000000000 ) ) ;
#5269=CARTESIAN_POINT ( 'NONE',  ( -17.45639740057859868, 21.16801284050013976, 101.0000000000000000 ) ) ;
#5270=ORIENTED_EDGE ( 'NONE', *, *, #8290, .F. ) ;
#5274=AXIS2_PLACEMENT_3D ( 'NONE', #4791, #14981, #8672 ) ;
#5296=ORIENTED_EDGE ( 'NONE', *, *, #14531, .F. ) ;
#5299=PLANE ( 'NONE',  #4919 ) ;
#5304=CARTESIAN_POINT ( 'NONE',  ( -14.89925740754307881, 13.32055945583976353, 101.0000000000000000 ) ) ;
#5311=ORIENTED_EDGE ( 'NONE', *, *, #210, .F. ) ;
#5314=CARTESIAN_POINT ( 'NONE',  ( 0.000000000000000000, 22.50000000000000000, 100.0000000000000000 ) ) ;
#5315=PLANE ( 'NONE',  #6815 ) ;
#5316=EDGE_CURVE ( 'NONE', #4152, #9378, #2553, .T. ) ;
#5336=DIRECTION ( 'NONE',  ( -1.000000000000000000, 0.000000000000000000, 0.000000000000000000 ) ) ;
#5337=DIRECTION ( 'NONE',  ( 0.000000000000000000, 0.000000000000000000, 1.000000000000000000 ) ) ;
#5344=DIRECTION ( 'NONE',  ( -0.000000000000000000, -0.000000000000000000, 1.000000000000000000 ) ) ;
#5346=CARTESIAN_POINT ( 'NONE',  ( 0.000000000000000000, 22.50000000000000000, 101.0000000000000000 ) ) ;
#5348=ADVANCED_FACE ( 'NONE', ( #2488 ), #16369, .T. ) ;
#5349=ORIENTED_EDGE ( 'NONE', *, *, #6117, .T. ) ;
#5351=ORIENTED_EDGE ( 'NONE', *, *, #5159, .F. ) ;
#5356=B_SPLINE_CURVE_WITH_KNOTS ( 'NONE', 3,
 ( #12713, #16285, #1482, #7724 ),
 .UNSPECIFIED., .F., .F.,
 ( 4, 4 ),
 ( 2.829004760659353259E-07, 0.001414802801989363968 ),
 .UNSPECIFIED. ) ;
#5358=DIRECTION ( 'NONE',  ( 0.000000000000000000, 0.000000000000000000, -1.000000000000000000 ) ) ;
#5362=LINE ( 'NONE', #11905, #5678 ) ;
#5373=ADVANCED_FACE ( 'NONE', ( #11238 ), #16216, .T. ) ;
#5385=ORIENTED_EDGE ( 'NONE', *, *, #16286, .F. ) ;
#5399=ORIENTED_EDGE ( 'NONE', *, *, #14670, .F. ) ;
#5401=AXIS2_PLACEMENT_3D ( 'NONE', #3313, #4495, #13370 ) ;
#5403=ORIENTED_EDGE ( 'NONE', *, *, #3603, .T. ) ;
#5405=ORIENTED_EDGE ( 'NONE', *, *, #1271, .F. ) ;
#5416=EDGE_CURVE ( 'NONE', #11934, #2664, #7412, .T. ) ;
#5422=ORIENTED_EDGE ( 'NONE', *, *, #10862, .F. ) ;
#5425=ORIENTED_EDGE ( 'NONE', *, *, #15590, .T. ) ;
#5429=PLANE ( 'NONE',  #1233 ) ;
#5433=PLANE ( 'NONE',  #3080 ) ;
#5441=VECTOR ( 'NONE', #9476, 999.9999999999998863 ) ;
#5460=EDGE_CURVE ( 'NONE', #2743, #9602, #10755, .T. ) ;
#5466=ORIENTED_EDGE ( 'NONE', *, *, #9680, .T. ) ;
#5469=CARTESIAN_POINT ( 'NONE',  ( -15.40544456622763470, 14.18301270189214947, 101.0000000000000000 ) ) ;
#5471=CIRCLE ( 'NONE', #4129, 16.50000000000000711 ) ;
#5472=CARTESIAN_POINT ( 'NONE',  ( 4.126043002969939977, 5.493361027597405410, 101.0000000000000000 ) ) ;
#5483=CIRCLE ( 'NONE', #13173, 17.50000000000000000 ) ;
#5491=CARTESIAN_POINT ( 'NONE',  ( -13.33959974903384627, 33.83821319854129683, 102.0000000000000142 ) ) ;
#5501=VECTOR ( 'NONE', #4780, 999.9999999999998863 ) ;
#5519=FACE_OUTER_BOUND ( 'NONE', #6364, .T. ) ;
#5521=CARTESIAN_POINT ( 'NONE',  ( 11.92169313911843354, 33.90715708214350599, 102.0000000000000142 ) ) ;
#5523=EDGE_CURVE ( 'NONE', #9777, #8525, #3673, .T. ) ;
#5533=EDGE_CURVE ( 'NONE', #16246, #9095, #12555, .T. ) ;
#5534=DIRECTION ( 'NONE',  ( -1.000000000000000000, 0.000000000000000000, 0.000000000000000000 ) ) ;
#5535=ORIENTED_EDGE ( 'NONE', *, *, #8930, .T. ) ;
#5559=CARTESIAN_POINT ( 'NONE',  ( 15.39925740754319605, 14.18658485962441240, 101.0000000000000000 ) ) ;
#5567=EDGE_CURVE ( 'NONE', #7399, #8881, #15926, .T. ) ;
#5586=CARTESIAN_POINT ( 'NONE',  ( -7.300484685133206142, 37.66786040234655530, 101.6666710451724214 ) ) ;
#5606=DIRECTION ( 'NONE',  ( -0.2079116908177665590, 0.9781476007338041345, 0.000000000000000000 ) ) ;
#5608=ADVANCED_FACE ( 'NONE', ( #9369 ), #13269, .T. ) ;
#5614=ADVANCED_FACE ( 'NONE', ( #4548 ), #7827, .T. ) ;
#5615=ADVANCED_FACE ( 'NONE', ( #14347 ), #4382, .T. ) ;
#5619=CARTESIAN_POINT ( 'NONE',  ( -6.661118525005218949, 38.69041383028340420, 101.0000000000000000 ) ) ;
#5640=EDGE_LOOP ( 'NONE', ( #4761, #3706, #14775, #10156 ) ) ;
#5642=B_SPLINE_CURVE_WITH_KNOTS ( 'NONE', 3,
 ( #2808, #1562, #6656, #11537 ),
 .UNSPECIFIED., .F., .F.,
 ( 4, 4 ),
 ( 0.01140363079879802566, 0.01281815069648909247 ),
 .UNSPECIFIED. ) ;
#5648=CARTESIAN_POINT ( 'NONE',  ( -8.880528407616480990, 25.91118970470954963, 102.0000000000000142 ) ) ;
#5649=DIRECTION ( 'NONE',  ( 0.4999999999999919509, 0.8660254037844432595, 0.000000000000000000 ) ) ;
#5652=DIRECTION ( 'NONE',  ( -0.7431448254773860285, -0.6691306063588672304, 0.000000000000000000 ) ) ;
#5653=AXIS2_PLACEMENT_3D ( 'NONE', #6568, #11626, #11701 ) ;
#5657=ORIENTED_EDGE ( 'NONE', *, *, #15569, .T. ) ;
#5661=VERTEX_POINT ( 'NONE', #6964 ) ;
#5666=ORIENTED_EDGE ( 'NONE', *, *, #2651, .F. ) ;
#5667=CARTESIAN_POINT ( 'NONE',  ( 16.79120288457601262, 27.43006142852259899, 101.0000000000000000 ) ) ;
#5673=DIRECTION ( 'NONE',  ( 1.224646799147353207E-16, -1.000000000000000000, 0.000000000000000000 ) ) ;
#5678=VECTOR ( 'NONE', #502, 1000.000000000000000 ) ;
#5685=EDGE_CURVE ( 'NONE', #7461, #960, #3050, .T. ) ;
#5688=AXIS2_PLACEMENT_3D ( 'NONE', #3810, #1218, #15022 ) ;
#5692=CARTESIAN_POINT ( 'NONE',  ( 4.320770838041294581, 30.97531352606685218, 101.0000000000000000 ) ) ;
#5703=ORIENTED_EDGE ( 'NONE', *, *, #8203, .T. ) ;
#5712=DIRECTION ( 'NONE',  ( -0.6691306063588569053, -0.7431448254773954654, 0.000000000000000000 ) ) ;
#5713=VECTOR ( 'NONE', #919, 1000.000000000000000 ) ;
#5723=ORIENTED_EDGE ( 'NONE', *, *, #6682, .T. ) ;
#5735=FACE_OUTER_BOUND ( 'NONE', #6214, .T. ) ;
#5741=EDGE_LOOP ( 'NONE', ( #6522, #5399, #11459, #264 ) ) ;
#5743=EDGE_CURVE ( 'NONE', #12158, #12941, #12185, .T. ) ;
#5748=FACE_OUTER_BOUND ( 'NONE', #15173, .T. ) ;
#5754=FACE_BOUND ( 'NONE', #8286, .T. ) ;
#5767=EDGE_LOOP ( 'NONE', ( #13077, #3216, #12293, #1305 ) ) ;
#5794=DIRECTION ( 'NONE',  ( 0.000000000000000000, 0.000000000000000000, 1.000000000000000000 ) ) ;
#5800=VERTEX_POINT ( 'NONE', #7290 ) ;
#5804=ORIENTED_EDGE ( 'NONE', *, *, #12255, .F. ) ;
#5805=LINE ( 'NONE', #12276, #8378 ) ;
#5806=CARTESIAN_POINT ( 'NONE',  ( 11.92169313911843354, 33.90715708214350599, 102.0000000000000142 ) ) ;
#5811=CARTESIAN_POINT ( 'NONE',  ( -16.50000000000000711, 22.50000000000000000, 102.0000000000000142 ) ) ;
#5817=EDGE_CURVE ( 'NONE', #12542, #16246, #2114, .T. ) ;
#5818=CARTESIAN_POINT ( 'NONE',  ( 0.000000000000000000, 22.50000000000000000, 102.0000000000000142 ) ) ;
#5819=B_SPLINE_CURVE_WITH_KNOTS ( 'NONE', 3,
 ( #11551, #15625, #7979, #8146 ),
 .UNSPECIFIED., .F., .F.,
 ( 4, 4 ),
 ( 2.829004760655812661E-07, 0.001414802801989366136 ),
 .UNSPECIFIED. ) ;
#5823=ORIENTED_EDGE ( 'NONE', *, *, #3585, .T. ) ;
#5824=ORIENTED_EDGE ( 'NONE', *, *, #8585, .F. ) ;
#5832=FILL_AREA_STYLE ('',( #3500 ) ) ;
#5850=B_SPLINE_CURVE_WITH_KNOTS ( 'NONE', 3,
 ( #11310, #8636, #62, #13709 ),
 .UNSPECIFIED., .F., .F.,
 ( 4, 4 ),
 ( 2.829004760671193191E-07, 0.001414802801989366787 ),
 .UNSPECIFIED. ) ;
#5852=DIRECTION ( 'NONE',  ( 0.4999999999999918954, 0.8660254037844433705, 0.000000000000000000 ) ) ;
#5859=DIRECTION ( 'NONE',  ( 0.000000000000000000, 0.000000000000000000, 1.000000000000000000 ) ) ;
#5866=EDGE_CURVE ( 'NONE', #8473, #11298, #1537, .T. ) ;
#5868=B_SPLINE_CURVE_WITH_KNOTS ( 'NONE', 3,
 ( #12052, #652, #15794, #1903 ),
 .UNSPECIFIED., .F., .F.,
 ( 4, 4 ),
 ( 2.829004760683457170E-07, 0.001414802801989366570 ),
 .UNSPECIFIED. ) ;
#5872=ORIENTED_EDGE ( 'NONE', *, *, #14727, .F. ) ;
#5876=CARTESIAN_POINT ( 'NONE',  ( 1.486087262401875941, 13.10364194761998213, 101.0000000000000000 ) ) ;
#5878=SHAPE_DEFINITION_REPRESENTATION ( #15551, #13393 ) ;
#5882=CARTESIAN_POINT ( 'NONE',  ( 0.5000000000000009992, 31.99999999999998579, 101.0000000000000000 ) ) ;
#5889=CARTESIAN_POINT ( 'NONE',  ( -4.320770838041405604, 30.97531352606679178, 101.0000000000000000 ) ) ;
#5890=FACE_OUTER_BOUND ( 'NONE', #13861, .T. ) ;
#5892=DIRECTION ( 'NONE',  ( -0.9945218953682744001, 0.1045284632676435066, 0.000000000000000000 ) ) ;
#5894=CARTESIAN_POINT ( 'NONE',  ( -2.464234863135557063, 13.31155363843772932, 102.0000000000000142 ) ) ;
#5899=CARTESIAN_POINT ( 'NONE',  ( 17.35186893731097868, 20.17349094513210161, 101.0000000000000000 ) ) ;
#5906=EDGE_LOOP ( 'NONE', ( #8289, #10871, #10080, #3879 ) ) ;
#5907=ORIENTED_EDGE ( 'NONE', *, *, #7051, .F. ) ;
#5912=CARTESIAN_POINT ( 'NONE',  ( 0.000000000000000000, 22.50000000000000000, 101.0000000000000000 ) ) ;
#5913=ORIENTED_EDGE ( 'NONE', *, *, #13293, .F. ) ;
#5931=VERTEX_POINT ( 'NONE', #5304 ) ;
#5945=EDGE_CURVE ( 'NONE', #13541, #589, #6198, .T. ) ;
#5969=VERTEX_POINT ( 'NONE', #6291 ) ;
#5970=ORIENTED_EDGE ( 'NONE', *, *, #5416, .T. ) ;
#5980=DIRECTION ( 'NONE',  ( 1.000000000000000000, 0.000000000000000000, 0.000000000000000000 ) ) ;
#5991=ORIENTED_EDGE ( 'NONE', *, *, #13801, .F. ) ;
#6005=EDGE_CURVE ( 'NONE', #9378, #4841, #110, .T. ) ;
#6016=CARTESIAN_POINT ( 'NONE',  ( 9.877534094663406705, 8.054089844915898411, 101.0000000000000000 ) ) ;
#6022=DIRECTION ( 'NONE',  ( 0.8660254037844362651, 0.5000000000000041078, 0.000000000000000000 ) ) ;
#6025=CARTESIAN_POINT ( 'NONE',  ( -16.34981105473763563, 20.27881147257167527, 102.0000000000000142 ) ) ;
#6042=ORIENTED_EDGE ( 'NONE', *, *, #7339, .T. ) ;
#6048=AXIS2_PLACEMENT_3D ( 'NONE', #12309, #9503, #9750 ) ;
#6057=ORIENTED_EDGE ( 'NONE', *, *, #7214, .F. ) ;
#6059=VECTOR ( 'NONE', #2558, 1000.000000000000227 ) ;
#6062=CARTESIAN_POINT ( 'NONE',  ( -12.67046914267499069, 34.58135802401869086, 102.0000000000000142 ) ) ;
#6067=EDGE_CURVE ( 'NONE', #10059, #3406, #4287, .T. ) ;
#6070=EDGE_CURVE ( 'NONE', #7551, #2664, #8185, .T. ) ;
#6075=CARTESIAN_POINT ( 'NONE',  ( -5.179451399590974781, 14.52044592729175321, 101.0000000000000000 ) ) ;
#6076=ORIENTED_EDGE ( 'NONE', *, *, #14840, .T. ) ;
#6077=ADVANCED_FACE ( 'NONE', ( #13251 ), #6947, .T. ) ;
#6081=VERTEX_POINT ( 'NONE', #597 ) ;
#6085=VERTEX_POINT ( 'NONE', #5692 ) ;
#6087=DIRECTION ( 'NONE',  ( 0.9781476007338069101, -0.2079116908177532363, 0.000000000000000000 ) ) ;
#6095=DIRECTION ( 'NONE',  ( -0.6691306063588671194, 0.7431448254773862505, 0.000000000000000000 ) ) ;
#6103=ORIENTED_EDGE ( 'NONE', *, *, #6195, .F. ) ;
#6107=LINE ( 'NONE', #14497, #10240 ) ;
#6117=EDGE_CURVE ( 'NONE', #9016, #14633, #3210, .T. ) ;
#6140=DIRECTION ( 'NONE',  ( 0.9510565162951544194, -0.3090169943749448422, 0.000000000000000000 ) ) ;
#6142=DIRECTION ( 'NONE',  ( 0.2079116908177531253, 0.9781476007338069101, 0.000000000000000000 ) ) ;
#6147=DIRECTION ( 'NONE',  ( -0.6691306063588673414, 0.7431448254773861395, 0.000000000000000000 ) ) ;
#6152=EDGE_LOOP ( 'NONE', ( #14448, #7574, #8604, #2900 ) ) ;
#6163=CARTESIAN_POINT ( 'NONE',  ( 0.000000000000000000, 22.50000000000000000, 101.0000000000000000 ) ) ;
#6164=DIRECTION ( 'NONE',  ( -1.000000000000000000, 0.000000000000000000, 0.000000000000000000 ) ) ;
#6166=PRESENTATION_STYLE_ASSIGNMENT (( #12642 ) ) ;
#6176=ORIENTED_EDGE ( 'NONE', *, *, #307, .T. ) ;
#6180=FACE_OUTER_BOUND ( 'NONE', #15341, .T. ) ;
#6195=EDGE_CURVE ( 'NONE', #13582, #3819, #11846, .T. ) ;
#6198=B_SPLINE_CURVE_WITH_KNOTS ( 'NONE', 3,
 ( #8771, #15245, #13833, #9103 ),
 .UNSPECIFIED., .F., .F.,
 ( 4, 4 ),
 ( 2.829004760702349710E-07, 0.001414802801989371557 ),
 .UNSPECIFIED. ) ;
#6203=ADVANCED_FACE ( 'NONE', ( #13172 ), #14330, .T. ) ;
#6214=EDGE_LOOP ( 'NONE', ( #15009, #15360, #8495, #3451 ) ) ;
#6225=CARTESIAN_POINT ( 'NONE',  ( 5.179451399591075145, 14.52044592729181538, 102.0000000000000142 ) ) ;
#6226=DIRECTION ( 'NONE',  ( 0.000000000000000000, 0.000000000000000000, -1.000000000000000000 ) ) ;
#6227=ORIENTED_EDGE ( 'NONE', *, *, #14153, .T. ) ;
#6238=CARTESIAN_POINT ( 'NONE',  ( -4.000000000000001776, 22.50000000000000000, 101.0000000000000000 ) ) ;
#6241=DIRECTION ( 'NONE',  ( 0.000000000000000000, 0.000000000000000000, -1.000000000000000000 ) ) ;
#6242=CARTESIAN_POINT ( 'NONE',  ( -17.35186893731094671, 20.17349094513186358, 102.0000000000000142 ) ) ;
#6244=CARTESIAN_POINT ( 'NONE',  ( 0.000000000000000000, 22.50000000000000000, 102.0000000000000142 ) ) ;
#6246=CARTESIAN_POINT ( 'NONE',  ( -9.881733417930727015, 8.048309972292139847, 101.0000000000000000 ) ) ;
#6249=VECTOR ( 'NONE', #14783, 1000.000000000000000 ) ;
#6264=DIRECTION ( 'NONE',  ( 0.4999999999999919509, 0.8660254037844432595, 0.000000000000000000 ) ) ;
#6269=CARTESIAN_POINT ( 'NONE',  ( 0.000000000000000000, 22.50000000000000000, 80.00000000000000000 ) ) ;
#6278=PRODUCT_DEFINITION_FORMATION_WITH_SPECIFIED_SOURCE ( 'ANY', '', #5220, .NOT_KNOWN. ) ;
#6282=EDGE_LOOP ( 'NONE', ( #13438, #11810, #14007, #4916 ) ) ;
#6288=AXIS2_PLACEMENT_3D ( 'NONE', #1921, #5852, #1086 ) ;
#6291=CARTESIAN_POINT ( 'NONE',  ( 6.725310538855729270, 29.22831317314791733, 102.0000000000000142 ) ) ;
#6298=VECTOR ( 'NONE', #8066, 1000.000000000000000 ) ;
#6304=CARTESIAN_POINT ( 'NONE',  ( 16.45433951800531247, 21.27333336794017171, 102.0000000000000142 ) ) ;
#6307=CIRCLE ( 'NONE', #12677, 17.50000000000000000 ) ;
#6316=CARTESIAN_POINT ( 'NONE',  ( 0.000000000000000000, 22.50000000000000000, 101.0000000000000000 ) ) ;
#6325=CARTESIAN_POINT ( 'NONE',  ( 0.000000000000000000, 22.50000000000000000, 102.0000000000000142 ) ) ;
#6327=ADVANCED_FACE ( 'NONE', ( #2017 ), #2352, .F. ) ;
#6331=DIRECTION ( 'NONE',  ( 1.000000000000000000, 0.000000000000000000, 0.000000000000000000 ) ) ;
#6343=DIRECTION ( 'NONE',  ( 0.000000000000000000, 0.000000000000000000, -1.000000000000000000 ) ) ;
#6344=EDGE_LOOP ( 'NONE', ( #5403, #4389 ) ) ;
#6357=DIRECTION ( 'NONE',  ( 0.000000000000000000, 0.000000000000000000, -1.000000000000000000 ) ) ;
#6363=EDGE_LOOP ( 'NONE', ( #2293, #3491 ) ) ;
#6364=EDGE_LOOP ( 'NONE', ( #12394, #2899, #3415, #1134 ) ) ;
#6366=VERTEX_POINT ( 'NONE', #12167 ) ;
#6371=CARTESIAN_POINT ( 'NONE',  ( -3.918041248536338728, 6.471932344328960696, 102.0000000000000142 ) ) ;
#6373=CARTESIAN_POINT ( 'NONE',  ( 17.45639740057861644, 21.16801284050037424, 102.0000000000000142 ) ) ;
#6374=EDGE_CURVE ( 'NONE', #10461, #10320, #2309, .T. ) ;
#6384=VERTEX_POINT ( 'NONE', #180 ) ;
#6393=CARTESIAN_POINT ( 'NONE',  ( 3.918041248536554555, 6.471932344329013098, 102.0000000000000142 ) ) ;
#6394=CARTESIAN_POINT ( 'NONE',  ( 19.48557158514982035, 33.75000000000009237, 101.0000000000000000 ) ) ;
#6395=CARTESIAN_POINT ( 'NONE',  ( -8.477241335952138357, 18.18301270189218855, 102.0000000000000142 ) ) ;
#6398=ORIENTED_EDGE ( 'NONE', *, *, #14511, .F. ) ;
#6403=CARTESIAN_POINT ( 'NONE',  ( 4.126043002969939977, 5.493361027597405410, 101.0000000000000000 ) ) ;
#6405=DIRECTION ( 'NONE',  ( 0.000000000000000000, 0.000000000000000000, -1.000000000000000000 ) ) ;
#6406=CARTESIAN_POINT ( 'NONE',  ( -0.4999999999999998890, 38.99242250247064590, 102.0000000000000142 ) ) ;
#6408=FACE_OUTER_BOUND ( 'NONE', #6814, .T. ) ;
#6413=DIRECTION ( 'NONE',  ( 0.000000000000000000, 0.000000000000000000, -1.000000000000000000 ) ) ;
#6416=ADVANCED_FACE ( 'NONE', ( #10335 ), #1094, .F. ) ;
#6421=DIRECTION ( 'NONE',  ( 0.000000000000000000, 0.000000000000000000, -1.000000000000000000 ) ) ;
#6435=CARTESIAN_POINT ( 'NONE',  ( -7.394441145214675437, 28.48516834767043093, 102.0000000000000142 ) ) ;
#6446=ORIENTED_EDGE ( 'NONE', *, *, #13630, .T. ) ;
#6455=CARTESIAN_POINT ( 'NONE',  ( -16.79799753235266735, 27.43226914341395783, 101.0000000000000000 ) ) ;
#6464=ORIENTED_EDGE ( 'NONE', *, *, #112, .T. ) ;
#6465=CARTESIAN_POINT ( 'NONE',  ( -12.66515988160626982, 34.57657754388018390, 101.0000000000000000 ) ) ;
#6466=CARTESIAN_POINT ( 'NONE',  ( -14.90544456622763470, 13.31698729810771376, 101.0000000000000000 ) ) ;
#6476=ORIENTED_EDGE ( 'NONE', *, *, #12382, .T. ) ;
#6481=EDGE_LOOP ( 'NONE', ( #7683, #1200, #10557, #1790 ) ) ;
#6482=ADVANCED_FACE ( 'NONE', ( #15143 ), #11420, .F. ) ;
#6483=PLANE ( 'NONE',  #8961 ) ;
#6486=FACE_OUTER_BOUND ( 'NONE', #2839, .T. ) ;
#6492=( NAMED_UNIT ( * ) PLANE_ANGLE_UNIT ( ) SI_UNIT ( $, .RADIAN. ) );
#6493=CARTESIAN_POINT ( 'NONE',  ( 10.09851121871635904, 9.451242543235769844, 102.0000000000000142 ) ) ;
#6495=DIRECTION ( 'NONE',  ( -0.9135454576426060846, 0.4067366430757887730, 0.000000000000000000 ) ) ;
#6502=ORIENTED_EDGE ( 'NONE', *, *, #12401, .T. ) ;
#6508=LINE ( 'NONE', #10412, #15809 ) ;
#6509=EDGE_CURVE ( 'NONE', #646, #9440, #4717, .T. ) ;
#6522=ORIENTED_EDGE ( 'NONE', *, *, #15590, .F. ) ;
#6526=EDGE_LOOP ( 'NONE', ( #1145, #10974, #1476, #5160 ) ) ;
#6527=ORIENTED_EDGE ( 'NONE', *, *, #3477, .F. ) ;
#6532=CARTESIAN_POINT ( 'NONE',  ( -3.078562342020560116, 5.611635739450979266, 101.3333374614808662 ) ) ;
#6550=AXIS2_PLACEMENT_3D ( 'NONE', #12160, #16152, #15978 ) ;
#6552=VECTOR ( 'NONE', #5017, 1000.000000000000000 ) ;
#6561=DIRECTION ( 'NONE',  ( 1.224646799147353207E-16, -1.000000000000000000, 0.000000000000000000 ) ) ;
#6568=CARTESIAN_POINT ( 'NONE',  ( 0.000000000000000000, 22.50000000000000000, 101.0000000000000000 ) ) ;
#6582=CARTESIAN_POINT ( 'NONE',  ( 17.35186893731097868, 20.17349094513210161, 101.0000000000000000 ) ) ;
#6587=LINE ( 'NONE', #13126, #3823 ) ;
#6594=ORIENTED_EDGE ( 'NONE', *, *, #915, .F. ) ;
#6603=DIRECTION ( 'NONE',  ( 0.8660254037844362651, 0.5000000000000041078, 0.000000000000000000 ) ) ;
#6605=LINE ( 'NONE', #12989, #2015 ) ;
#6609=CARTESIAN_POINT ( 'NONE',  ( -4.320770838041405604, 30.97531352606679178, 101.0000000000000000 ) ) ;
#6620=CARTESIAN_POINT ( 'NONE',  ( 7.732050807568878525, 22.50000000000000000, 102.0000000000000142 ) ) ;
#6633=EDGE_CURVE ( 'NONE', #9602, #1101, #579, .T. ) ;
#6634=EDGE_CURVE ( 'NONE', #11447, #2664, #6772, .T. ) ;
#6637=ORIENTED_EDGE ( 'NONE', *, *, #127, .T. ) ;
#6643=CARTESIAN_POINT ( 'NONE',  ( -14.53285685708567421, 14.68680145065682474, 102.0000000000000142 ) ) ;
#6647=ADVANCED_FACE ( 'NONE', ( #16142 ), #3507, .F. ) ;
#6652=PLANE ( 'NONE',  #11484 ) ;
#6653=ORIENTED_EDGE ( 'NONE', *, *, #10082, .T. ) ;
#6656=CARTESIAN_POINT ( 'NONE',  ( -0.4999999999999998890, 39.32590460608501104, 101.6666710454654208 ) ) ;
#6658=ORIENTED_EDGE ( 'NONE', *, *, #3489, .T. ) ;
#6665=CARTESIAN_POINT ( 'NONE',  ( -7.732050807568878525, 22.50000000000000000, 102.0000000000000142 ) ) ;
#6678=CARTESIAN_POINT ( 'NONE',  ( 0.000000000000000000, 22.50000000000000000, 101.0000000000000000 ) ) ;
#6682=EDGE_CURVE ( 'NONE', #9526, #11778, #8076, .T. ) ;
#6691=LINE ( 'NONE', #11739, #1772 ) ;
#6695=CYLINDRICAL_SURFACE ( 'NONE', #3274, 17.50000000000000000 ) ;
#6714=ORIENTED_EDGE ( 'NONE', *, *, #6634, .F. ) ;
#6730=LINE ( 'NONE', #4054, #10693 ) ;
#6731=VERTEX_POINT ( 'NONE', #11074 ) ;
#6734=B_SPLINE_CURVE_WITH_KNOTS ( 'NONE', 3,
 ( #6016, #2249, #2166, #7260 ),
 .UNSPECIFIED., .F., .F.,
 ( 4, 4 ),
 ( 2.829004760673572825E-07, 0.001414802801989366570 ),
 .UNSPECIFIED. ) ;
#6738=ORIENTED_EDGE ( 'NONE', *, *, #10776, .T. ) ;
#6748=DIRECTION ( 'NONE',  ( 0.000000000000000000, 0.000000000000000000, -1.000000000000000000 ) ) ;
#6751=FACE_OUTER_BOUND ( 'NONE', #10386, .T. ) ;
#6753=LINE ( 'NONE', #3996, #12405 ) ;
#6755=CARTESIAN_POINT ( 'NONE',  ( -8.477241335952138357, 18.18301270189218855, 101.0000000000000000 ) ) ;
#6756=CARTESIAN_POINT ( 'NONE',  ( -16.45433951800529826, 21.27333336793995144, 102.0000000000000142 ) ) ;
#6760=ORIENTED_EDGE ( 'NONE', *, *, #7347, .T. ) ;
#6770=CARTESIAN_POINT ( 'NONE',  ( 7.732050807568878525, 22.50000000000000000, 100.0000000000000000 ) ) ;
#6772=LINE ( 'NONE', #1674, #14693 ) ;
#6779=LINE ( 'NONE', #11912, #10445 ) ;
#6780=ORIENTED_EDGE ( 'NONE', *, *, #9277, .F. ) ;
#6782=ORIENTED_EDGE ( 'NONE', *, *, #3477, .T. ) ;
#6791=CARTESIAN_POINT ( 'NONE',  ( -9.289494224341229511, 8.863457290943159705, 102.0000000000000142 ) ) ;
#6798=ORIENTED_EDGE ( 'NONE', *, *, #12723, .F. ) ;
#6812=CIRCLE ( 'NONE', #10522, 16.50000000000000711 ) ;
#6814=EDGE_LOOP ( 'NONE', ( #5349, #12275, #13461, #3236 ) ) ;
#6815=AXIS2_PLACEMENT_3D ( 'NONE', #1548, #6883, #7786 ) ;
#6819=EDGE_LOOP ( 'NONE', ( #15461, #5970, #6714, #13681 ) ) ;
#6821=DIRECTION ( 'NONE',  ( -0.3090169943749574988, 0.9510565162951503115, 0.000000000000000000 ) ) ;
#6823=LINE ( 'NONE', #7054, #3342 ) ;
#6827=CIRCLE ( 'NONE', #8392, 16.50000000000000711 ) ;
#6828=CIRCLE ( 'NONE', #15837, 2.000000000000001776 ) ;
#6848=EDGE_LOOP ( 'NONE', ( #14452, #15878, #14971, #14513 ) ) ;
#6851=FACE_OUTER_BOUND ( 'NONE', #3125, .T. ) ;
#6855=B_SPLINE_CURVE_WITH_KNOTS ( 'NONE', 3,
 ( #15279, #16378, #10312, #7727 ),
 .UNSPECIFIED., .F., .F.,
 ( 4, 4 ),
 ( 2.829004760695596740E-07, 0.001414802801989369606 ),
 .UNSPECIFIED. ) ;
#6856=VECTOR ( 'NONE', #14627, 1000.000000000000227 ) ;
#6868=CARTESIAN_POINT ( 'NONE',  ( -3.147895402235901141, 5.285449336779595164, 101.0000000000000000 ) ) ;
#6881=CIRCLE ( 'NONE', #16163, 17.50000000000000000 ) ;
#6882=ORIENTED_EDGE ( 'NONE', *, *, #10785, .T. ) ;
#6883=DIRECTION ( 'NONE',  ( 0.000000000000000000, 0.000000000000000000, -1.000000000000000000 ) ) ;
#6896=ORIENTED_EDGE ( 'NONE', *, *, #10486, .F. ) ;
#6899=CARTESIAN_POINT ( 'NONE',  ( 0.000000000000000000, 22.50000000000000000, 101.0000000000000000 ) ) ;
#6900=CARTESIAN_POINT ( 'NONE',  ( 0.000000000000000000, 22.50000000000000000, 101.0000000000000000 ) ) ;
#6904=DIRECTION ( 'NONE',  ( 1.000000000000000000, 0.000000000000000000, 0.000000000000000000 ) ) ;
#6905=DIRECTION ( 'NONE',  ( 0.000000000000000000, 0.000000000000000000, -1.000000000000000000 ) ) ;
#6919=LINE ( 'NONE', #328, #13195 ) ;
#6923=CARTESIAN_POINT ( 'NONE',  ( 0.000000000000000000, 22.50000000000000000, 102.0000000000000142 ) ) ;
#6947=PLANE ( 'NONE',  #15273 ) ;
#6952=EDGE_CURVE ( 'NONE', #9016, #14534, #9989, .T. ) ;
#6958=EDGE_CURVE ( 'NONE', #4332, #11934, #14674, .T. ) ;
#6960=PLANE ( 'NONE',  #413 ) ;
#6964=CARTESIAN_POINT ( 'NONE',  ( -0.4999999999999990563, 31.99999999999998579, 101.0000000000000000 ) ) ;
#6976=DIRECTION ( 'NONE',  ( 1.000000000000000000, 0.000000000000000000, 0.000000000000000000 ) ) ;
#6978=LINE ( 'NONE', #5648, #12034 ) ;
#6980=LINE ( 'NONE', #637, #11272 ) ;
#6982=CIRCLE ( 'NONE', #8302, 17.50000000000000000 ) ;
#7006=CARTESIAN_POINT ( 'NONE',  ( 4.127528389677815213, 5.486372832567310454, 101.0000000000000000 ) ) ;
#7037=ADVANCED_FACE ( 'NONE', ( #6751 ), #12883, .F. ) ;
#7038=LINE ( 'NONE', #11769, #13170 ) ;
#7047=VERTEX_POINT ( 'NONE', #2826 ) ;
#7048=ORIENTED_EDGE ( 'NONE', *, *, #14177, .F. ) ;
#7051=EDGE_CURVE ( 'NONE', #14108, #13278, #4798, .T. ) ;
#7054=CARTESIAN_POINT ( 'NONE',  ( -6.725310538855818976, 29.22831317314782851, 101.0000000000000000 ) ) ;
#7061=LINE ( 'NONE', #731, #3563 ) ;
#7062=LINE ( 'NONE', #5899, #1515 ) ;
#7065=CARTESIAN_POINT ( 'NONE',  ( -7.164845293664018122, 37.36320934111677161, 102.0000000000000142 ) ) ;
#7071=ORIENTED_EDGE ( 'NONE', *, *, #3249, .F. ) ;
#7076=CARTESIAN_POINT ( 'NONE',  ( -7.164845293664018122, 37.36320934111677161, 102.0000000000000142 ) ) ;
#7077=LINE ( 'NONE', #14615, #6249 ) ;
#7078=CIRCLE ( 'NONE', #12108, 17.50000000000000000 ) ;
#7088=EDGE_CURVE ( 'NONE', #12113, #562, #6587, .T. ) ;
#7092=CARTESIAN_POINT ( 'NONE',  ( 0.5000000000000009992, 31.99999999999998579, 102.0000000000000142 ) ) ;
#7096=CIRCLE ( 'NONE', #10271, 16.50000000000000711 ) ;
#7124=DIRECTION ( 'NONE',  ( 0.2079116908177531531, 0.9781476007338069101, 0.000000000000000000 ) ) ;
#7130=ADVANCED_FACE ( 'NONE', ( #11796 ), #15453, .F. ) ;
#7133=ORIENTED_EDGE ( 'NONE', *, *, #15667, .T. ) ;
#7147=LINE ( 'NONE', #12459, #2834 ) ;
#7149=CARTESIAN_POINT ( 'NONE',  ( -9.500222237632405253, 22.00424054664139817, 102.0000000000000142 ) ) ;
#7161=PLANE ( 'NONE',  #11343 ) ;
#7170=CARTESIAN_POINT ( 'NONE',  ( 2.267949192431125027, 22.50000000000000000, 100.0000000000000000 ) ) ;
#7198=PLANE ( 'NONE',  #15820 ) ;
#7211=VERTEX_POINT ( 'NONE', #8467 ) ;
#7214=EDGE_CURVE ( 'NONE', #13541, #3156, #12314, .T. ) ;
#7216=CARTESIAN_POINT ( 'NONE',  ( -14.90544456622763470, 13.31698729810771376, 101.0000000000000000 ) ) ;
#7234=VERTEX_POINT ( 'NONE', #4404 ) ;
#7236=CARTESIAN_POINT ( 'NONE',  ( -9.881733417930727015, 8.048309972292139847, 102.0000000000000142 ) ) ;
#7241=DIRECTION ( 'NONE',  ( 0.000000000000000000, 0.000000000000000000, 1.000000000000000000 ) ) ;
#7243=DIRECTION ( 'NONE',  ( -0.5877852522924689183, -0.8090169943749505599, 0.000000000000000000 ) ) ;
#7247=CIRCLE ( 'NONE', #5653, 17.50000000000000000 ) ;
#7249=EDGE_CURVE ( 'NONE', #14171, #566, #3148, .T. ) ;
#7253=B_SPLINE_CURVE_WITH_KNOTS ( 'NONE', 3,
 ( #12418, #1007, #4783, #13644 ),
 .UNSPECIFIED., .F., .F.,
 ( 4, 4 ),
 ( 2.829004760673920638E-07, 0.001414802801989366136 ),
 .UNSPECIFIED. ) ;
#7259=CONICAL_SURFACE ( 'NONE', #9112, 16.50000000000000711, 0.7853981633974447263 ) ;
#7260=CARTESIAN_POINT ( 'NONE',  ( 9.289494224341416029, 8.863457290943287603, 102.0000000000000142 ) ) ;
#7263=B_SPLINE_CURVE_WITH_KNOTS ( 'NONE', 3,
 ( #5142, #5067, #14256, #2876 ),
 .UNSPECIFIED., .F., .F.,
 ( 4, 4 ),
 ( 2.829004760695596740E-07, 0.001414802801989370690 ),
 .UNSPECIFIED. ) ;
#7266=EDGE_CURVE ( 'NONE', #605, #7385, #13908, .T. ) ;
#7284=VECTOR ( 'NONE', #7636, 1000.000000000000000 ) ;
#7290=CARTESIAN_POINT ( 'NONE',  ( -2.939893647802529930, 6.264020653511205516, 102.0000000000000142 ) ) ;
#7296=ORIENTED_EDGE ( 'NONE', *, *, #7266, .F. ) ;
#7300=ORIENTED_EDGE ( 'NONE', *, *, #2598, .F. ) ;
#7303=PLANE ( 'NONE',  #14730 ) ;
#7313=CARTESIAN_POINT ( 'NONE',  ( 3.147895402236133400, 5.285449336779636909, 101.0000000000000000 ) ) ;
#7317=VERTEX_POINT ( 'NONE', #13367 ) ;
#7319=ORIENTED_EDGE ( 'NONE', *, *, #9318, .T. ) ;
#7323=ORIENTED_EDGE ( 'NONE', *, *, #14511, .T. ) ;
#7325=( LENGTH_UNIT ( ) NAMED_UNIT ( * ) SI_UNIT ( .MILLI., .METRE. ) );
#7335=DIRECTION ( 'NONE',  ( 0.9781476007338041345, 0.2079116908177665313, 0.000000000000000000 ) ) ;
#7339=EDGE_CURVE ( 'NONE', #11991, #8154, #6980, .T. ) ;
#7344=TOROIDAL_SURFACE ( 'NONE', #8393, 2.267949192431125027, 2.000000000000000000 ) ;
#7346=CARTESIAN_POINT ( 'NONE',  ( 4.320770838041294581, 30.97531352606685218, 102.0000000000000142 ) ) ;
#7347=EDGE_CURVE ( 'NONE', #7211, #10911, #7061, .T. ) ;
#7348=EDGE_LOOP ( 'NONE', ( #3474, #6782, #4373, #13782 ) ) ;
#7352=DIRECTION ( 'NONE',  ( 1.000000000000000000, 0.000000000000000000, 0.000000000000000000 ) ) ;
#7362=DIRECTION ( 'NONE',  ( 0.1045284632676436315, 0.9945218953682742891, 0.000000000000000000 ) ) ;
#7372=VERTEX_POINT ( 'NONE', #2060 ) ;
#7373=DIRECTION ( 'NONE',  ( 0.5877852522924688072, 0.8090169943749505599, 0.000000000000000000 ) ) ;
#7383=VERTEX_POINT ( 'NONE', #7149 ) ;
#7385=VERTEX_POINT ( 'NONE', #12210 ) ;
#7394=PLANE ( 'NONE',  #9401 ) ;
#7399=VERTEX_POINT ( 'NONE', #12617 ) ;
#7409=CARTESIAN_POINT ( 'NONE',  ( -6.725310538855818976, 29.22831317314782851, 101.0000000000000000 ) ) ;
#7412=LINE ( 'NONE', #9119, #707 ) ;
#7416=ADVANCED_FACE ( 'NONE', ( #5077 ), #5166, .T. ) ;
#7423=VERTEX_POINT ( 'NONE', #2467 ) ;
#7443=ORIENTED_EDGE ( 'NONE', *, *, #14840, .F. ) ;
#7444=EDGE_CURVE ( 'NONE', #4152, #646, #50, .T. ) ;
#7446=ORIENTED_EDGE ( 'NONE', *, *, #15400, .F. ) ;
#7461=VERTEX_POINT ( 'NONE', #6393 ) ;
#7463=CARTESIAN_POINT ( 'NONE',  ( 16.78599477205478863, 21.23847499609146183, 101.6666710451724214 ) ) ;
#7465=CARTESIAN_POINT ( 'NONE',  ( 8.880528407616436581, 25.91118970470966687, 101.0000000000000000 ) ) ;
#7467=ADVANCED_FACE ( 'NONE', ( #5153 ), #7394, .T. ) ;
#7469=DIRECTION ( 'NONE',  ( -0.7431448254773860285, -0.6691306063588672304, 0.000000000000000000 ) ) ;
#7470=CARTESIAN_POINT ( 'NONE',  ( -7.732050807568878525, 22.50000000000000000, 100.0000000000000000 ) ) ;
#7478=DIRECTION ( 'NONE',  ( 1.000000000000000000, 0.000000000000000000, 0.000000000000000000 ) ) ;
#7484=CARTESIAN_POINT ( 'NONE',  ( -9.500222237632405253, 22.00424054664139817, 101.0000000000000000 ) ) ;
#7485=DIRECTION ( 'NONE',  ( -0.4067366430757887175, -0.9135454576426059736, 0.000000000000000000 ) ) ;
#7489=CARTESIAN_POINT ( 'NONE',  ( 6.386939227490392668, 38.07459704542245049, 101.6666710451724214 ) ) ;
#7496=EDGE_LOOP ( 'NONE', ( #4554, #6527, #3977, #5703 ) ) ;
#7507=CARTESIAN_POINT ( 'NONE',  ( 9.189545401991395579, 24.96013318841451678, 101.0000000000000000 ) ) ;
#7512=B_SPLINE_CURVE_WITH_KNOTS ( 'NONE', 3,
 ( #10953, #15938, #2207, #5806 ),
 .UNSPECIFIED., .F., .F.,
 ( 4, 4 ),
 ( 2.829004760702349710E-07, 0.001414802801989369606 ),
 .UNSPECIFIED. ) ;
#7530=ADVANCED_FACE ( 'NONE', ( #1054 ), #3654, .T. ) ;
#7536=LINE ( 'NONE', #10040, #7863 ) ;
#7541=CARTESIAN_POINT ( 'NONE',  ( 0.000000000000000000, 22.50000000000000000, 102.0000000000000142 ) ) ;
#7546=AXIS2_PLACEMENT_3D ( 'NONE', #3402, #9806, #5980 ) ;
#7551=VERTEX_POINT ( 'NONE', #6225 ) ;
#7572=CARTESIAN_POINT ( 'NONE',  ( 0.000000000000000000, 22.50000000000000000, 101.0000000000000000 ) ) ;
#7574=ORIENTED_EDGE ( 'NONE', *, *, #8290, .T. ) ;
#7595=VECTOR ( 'NONE', #8954, 1000.000000000000114 ) ;
#7598=ORIENTED_EDGE ( 'NONE', *, *, #5256, .T. ) ;
#7607=CARTESIAN_POINT ( 'NONE',  ( -21.39877161664088234, 15.54711762656345897, 101.0000000000000000 ) ) ;
#7611=DIRECTION ( 'NONE',  ( -0.9135454576426004225, -0.4067366430758009854, 0.000000000000000000 ) ) ;
#7619=DIRECTION ( 'NONE',  ( 0.000000000000000000, -0.000000000000000000, 1.000000000000000000 ) ) ;
#7636=DIRECTION ( 'NONE',  ( -0.000000000000000000, -0.000000000000000000, -1.000000000000000000 ) ) ;
#7642=ORIENTED_EDGE ( 'NONE', *, *, #8744, .F. ) ;
#7643=CARTESIAN_POINT ( 'NONE',  ( -8.477241335952138357, 18.18301270189218855, 101.0000000000000000 ) ) ;
#7645=ORIENTED_EDGE ( 'NONE', *, *, #15916, .F. ) ;
#7652=LINE ( 'NONE', #6242, #15489 ) ;
#7659=ORIENTED_EDGE ( 'NONE', *, *, #3464, .T. ) ;
#7662=EDGE_CURVE ( 'NONE', #1769, #5969, #15353, .T. ) ;
#7677=AXIS2_PLACEMENT_3D ( 'NONE', #8051, #6905, #7893 ) ;
#7683=ORIENTED_EDGE ( 'NONE', *, *, #14127, .F. ) ;
#7686=ORIENTED_EDGE ( 'NONE', *, *, #13835, .T. ) ;
#7695=DIRECTION ( 'NONE',  ( 0.9510565162951544194, -0.3090169943749448422, 0.000000000000000000 ) ) ;
#7714=DIRECTION ( 'NONE',  ( 0.000000000000000000, -0.000000000000000000, 1.000000000000000000 ) ) ;
#7724=CARTESIAN_POINT ( 'NONE',  ( 7.164845293663816506, 37.36320934111687109, 102.0000000000000142 ) ) ;
#7726=DIRECTION ( 'NONE',  ( 1.000000000000000000, 0.000000000000000000, 0.000000000000000000 ) ) ;
#7727=CARTESIAN_POINT ( 'NONE',  ( -16.34981105473763563, 20.27881147257167527, 102.0000000000000142 ) ) ;
#7730=CARTESIAN_POINT ( 'NONE',  ( 5.988468393966018155, 15.10823117958429584, 102.0000000000000142 ) ) ;
#7731=SURFACE_STYLE_FILL_AREA ( #11471 ) ;
#7732=CARTESIAN_POINT ( 'NONE',  ( 10.68655108903834794, 8.641875097208380652, 101.0000000000000000 ) ) ;
#7744=VERTEX_POINT ( 'NONE', #11435 ) ;
#7763=ADVANCED_FACE ( 'NONE', ( #5133 ), #9939, .F. ) ;
#7769=CARTESIAN_POINT ( 'NONE',  ( -3.407225380398804404, 31.38205016914259105, 101.0000000000000000 ) ) ;
#7774=VECTOR ( 'NONE', #14270, 999.9999999999998863 ) ;
#7781=VERTEX_POINT ( 'NONE', #11273 ) ;
#7783=VECTOR ( 'NONE', #10944, 1000.000000000000000 ) ;
#7785=LINE ( 'NONE', #1705, #12939 ) ;
#7786=DIRECTION ( 'NONE',  ( 0.8090169943749426773, 0.5877852522924797984, 0.000000000000000000 ) ) ;
#7787=ADVANCED_FACE ( 'NONE', ( #2614 ), #4968, .T. ) ;
#7807=DIRECTION ( 'NONE',  ( 1.000000000000000000, 0.000000000000000000, 0.000000000000000000 ) ) ;
#7808=DIRECTION ( 'NONE',  ( -0.000000000000000000, 0.000000000000000000, 1.000000000000000000 ) ) ;
#7815=CARTESIAN_POINT ( 'NONE',  ( 4.320770838041294581, 30.97531352606685218, 102.0000000000000142 ) ) ;
#7817=CIRCLE ( 'NONE', #629, 17.50000000000000000 ) ;
#7824=ORIENTED_EDGE ( 'NONE', *, *, #13293, .T. ) ;
#7826=CARTESIAN_POINT ( 'NONE',  ( -6.000000000000001776, 22.50000000000000000, 101.0000000000000000 ) ) ;
#7827=CONICAL_SURFACE ( 'NONE', #10495, 16.50000000000000711, 0.7853981633974447263 ) ;
#7830=DIRECTION ( 'NONE',  ( 0.000000000000000000, -0.000000000000000000, 1.000000000000000000 ) ) ;
#7841=ORIENTED_EDGE ( 'NONE', *, *, #11329, .F. ) ;
#7852=CIRCLE ( 'NONE', #12894, 17.50000000000000000 ) ;
#7860=ORIENTED_EDGE ( 'NONE', *, *, #16301, .F. ) ;
#7863=VECTOR ( 'NONE', #8780, 1000.000000000000000 ) ;
#7867=DIRECTION ( 'NONE',  ( 0.000000000000000000, 0.000000000000000000, -1.000000000000000000 ) ) ;
#7885=AXIS2_PLACEMENT_3D ( 'NONE', #14604, #12285, #14527 ) ;
#7888=VECTOR ( 'NONE', #10559, 1000.000000000000000 ) ;
#7889=CARTESIAN_POINT ( 'NONE',  ( -9.151574469205250750, 1.945227203041358877, 101.0000000000000000 ) ) ;
#7893=DIRECTION ( 'NONE',  ( -1.000000000000000000, 0.000000000000000000, 0.000000000000000000 ) ) ;
#7896=DIRECTION ( 'NONE',  ( -0.6691306063588567943, -0.7431448254773955764, 0.000000000000000000 ) ) ;
#7907=VERTEX_POINT ( 'NONE', #13005 ) ;
#7910=CARTESIAN_POINT ( 'NONE',  ( 7.574663982647604321, 38.28367718720770796, 101.0000000000000000 ) ) ;
#7913=CARTESIAN_POINT ( 'NONE',  ( -7.574663982647817484, 38.28367718720760138, 101.0000000000000000 ) ) ;
#7924=VERTEX_POINT ( 'NONE', #14244 ) ;
#7931=DIRECTION ( 'NONE',  ( 1.000000000000000000, 0.000000000000000000, 0.000000000000000000 ) ) ;
#7937=CARTESIAN_POINT ( 'NONE',  ( -9.485510086921518536, 8.593664601562084115, 101.6666710451724214 ) ) ;
#7941=EDGE_CURVE ( 'NONE', #16202, #14151, #11802, .T. ) ;
#7951=EDGE_CURVE ( 'NONE', #2544, #12958, #7817, .T. ) ;
#7968=ADVANCED_FACE ( 'NONE', ( #14325 ), #5299, .T. ) ;
#7979=CARTESIAN_POINT ( 'NONE',  ( -16.15689471564406432, 27.22396221095493729, 101.6666710451724214 ) ) ;
#7981=LINE ( 'NONE', #5269, #4327 ) ;
#7984=ORIENTED_EDGE ( 'NONE', *, *, #11252, .T. ) ;
#7985=EDGE_LOOP ( 'NONE', ( #12469, #11146, #12626, #15934 ) ) ;
#7987=LINE ( 'NONE', #13224, #4719 ) ;
#7989=VERTEX_POINT ( 'NONE', #6620 ) ;
#7996=DIRECTION ( 'NONE',  ( 0.000000000000000000, 0.000000000000000000, -1.000000000000000000 ) ) ;
#7999=LINE ( 'NONE', #13073, #12387 ) ;
#8005=ORIENTED_EDGE ( 'NONE', *, *, #11699, .T. ) ;
#8039=CONICAL_SURFACE ( 'NONE', #12565, 16.50000000000000711, 0.7853981633974447263 ) ;
#8046=DIRECTION ( 'NONE',  ( 0.7431448254773955764, -0.6691306063588567943, 0.000000000000000000 ) ) ;
#8051=CARTESIAN_POINT ( 'NONE',  ( 0.000000000000000000, 22.50000000000000000, 102.0000000000000142 ) ) ;
#8052=VECTOR ( 'NONE', #15774, 1000.000000000000000 ) ;
#8056=CARTESIAN_POINT ( 'NONE',  ( 16.47405064338586200, 27.32701241865550656, 101.3333374614808662 ) ) ;
#8063=ORIENTED_EDGE ( 'NONE', *, *, #10590, .F. ) ;
#8066=DIRECTION ( 'NONE',  ( -0.000000000000000000, -0.000000000000000000, 1.000000000000000000 ) ) ;
#8069=DIRECTION ( 'NONE',  ( 0.1045284632676570929, -0.9945218953682730678, 0.000000000000000000 ) ) ;
#8076=CIRCLE ( 'NONE', #8871, 2.000000000000000000 ) ;
#8082=DIRECTION ( 'NONE',  ( -1.000000000000000000, 0.000000000000000000, 0.000000000000000000 ) ) ;
#8086=VERTEX_POINT ( 'NONE', #11830 ) ;
#8089=AXIS2_PLACEMENT_3D ( 'NONE', #1251, #6343, #11409 ) ;
#8095=DIRECTION ( 'NONE',  ( 1.000000000000000000, 0.000000000000000000, 0.000000000000000000 ) ) ;
#8111=MECHANICAL_DESIGN_GEOMETRIC_PRESENTATION_REPRESENTATION('',(#12359),#8644);
#8117=VECTOR ( 'NONE', #137, 999.9999999999998863 ) ;
#8126=EDGE_LOOP ( 'NONE', ( #918, #6760, #16123, #15706 ) ) ;
#8131=CARTESIAN_POINT ( 'NONE',  ( 0.000000000000000000, 22.50000000000000000, 102.0000000000000142 ) ) ;
#8140=CARTESIAN_POINT ( 'NONE',  ( 3.407225380398686276, 31.38205016914263723, 101.0000000000000000 ) ) ;
#8146=CARTESIAN_POINT ( 'NONE',  ( -15.83973438765502451, 27.12091057352761325, 102.0000000000000142 ) ) ;
#8148=CARTESIAN_POINT ( 'NONE',  ( -11.92169313911859341, 33.90715708214334256, 102.0000000000000142 ) ) ;
#8149=ORIENTED_EDGE ( 'NONE', *, *, #16173, .T. ) ;
#8153=VERTEX_POINT ( 'NONE', #11231 ) ;
#8154=VERTEX_POINT ( 'NONE', #9898 ) ;
#8159=EDGE_LOOP ( 'NONE', ( #7133, #11353, #12961, #15155, #16307, #12539, #13379, #16396, #11129, #15997, #10120, #13435, #6076, #6738, #3493, #4313, #9887, #1822 ) ) ;
#8160=DIRECTION ( 'NONE',  ( 0.4067366430758010964, -0.9135454576426004225, 0.000000000000000000 ) ) ;
#8164=FACE_OUTER_BOUND ( 'NONE', #8903, .T. ) ;
#8185=LINE ( 'NONE', #15492, #12101 ) ;
#8192=VERTEX_POINT ( 'NONE', #6238 ) ;
#8195=B_SPLINE_CURVE_WITH_KNOTS ( 'NONE', 3,
 ( #2793, #12946, #1550, #6643 ),
 .UNSPECIFIED., .F., .F.,
 ( 4, 4 ),
 ( 2.829004760673920638E-07, 0.001414802801989366136 ),
 .UNSPECIFIED. ) ;
#8202=DIRECTION ( 'NONE',  ( -0.8660254037844433705, 0.4999999999999918399, 0.000000000000000000 ) ) ;
#8203=EDGE_CURVE ( 'NONE', #7781, #6366, #9740, .T. ) ;
#8210=EDGE_LOOP ( 'NONE', ( #14655, #7860, #9872, #9546 ) ) ;
#8212=CARTESIAN_POINT ( 'NONE',  ( 0.5000000000000009992, 31.99999999999998579, 102.0000000000000142 ) ) ;
#8213=CARTESIAN_POINT ( 'NONE',  ( -12.67046914267499069, 34.58135802401869086, 101.0000000000000000 ) ) ;
#8232=ORIENTED_EDGE ( 'NONE', *, *, #1475, .T. ) ;
#8236=EDGE_LOOP ( 'NONE', ( #14429, #12511, #3300, #2416 ) ) ;
#8243=CARTESIAN_POINT ( 'NONE',  ( 16.48898053797764973, 28.38332565970932819, 101.0000000000000000 ) ) ;
#8244=CARTESIAN_POINT ( 'NONE',  ( -16.72075857324118786, 7.444561356925489370, 101.0000000000000000 ) ) ;
#8246=CARTESIAN_POINT ( 'NONE',  ( 9.289494224341416029, 8.863457290943287603, 102.0000000000000142 ) ) ;
#8256=FACE_OUTER_BOUND ( 'NONE', #6363, .T. ) ;
#8275=VERTEX_POINT ( 'NONE', #4040 ) ;
#8286=EDGE_LOOP ( 'NONE', ( #4924, #4058 ) ) ;
#8289=ORIENTED_EDGE ( 'NONE', *, *, #10208, .F. ) ;
#8290=EDGE_CURVE ( 'NONE', #14428, #8817, #7263, .T. ) ;
#8302=AXIS2_PLACEMENT_3D ( 'NONE', #6316, #890, #2471 ) ;
#8304=DIRECTION ( 'NONE',  ( 0.8090169943749504489, -0.5877852522924689183, 0.000000000000000000 ) ) ;
#8305=EDGE_LOOP ( 'NONE', ( #2146, #162, #2150, #10968 ) ) ;
#8308=EDGE_LOOP ( 'NONE', ( #9529, #14514, #8843, #9809 ) ) ;
#8315=DIRECTION ( 'NONE',  ( 0.7431448254773955764, -0.6691306063588567943, 0.000000000000000000 ) ) ;
#8323=DIRECTION ( 'NONE',  ( 0.000000000000000000, 0.000000000000000000, -1.000000000000000000 ) ) ;
#8337=AXIS2_PLACEMENT_3D ( 'NONE', #14201, #7896, #12971 ) ;
#8338=CARTESIAN_POINT ( 'NONE',  ( 0.000000000000000000, 22.50000000000000000, 102.0000000000000142 ) ) ;
#8357=DIRECTION ( 'NONE',  ( -0.9510565162951503115, -0.3090169943749574988, 0.000000000000000000 ) ) ;
#8358=CIRCLE ( 'NONE', #1182, 17.50000000000000000 ) ;
#8366=ORIENTED_EDGE ( 'NONE', *, *, #2468, .F. ) ;
#8368=CIRCLE ( 'NONE', #5203, 16.50000000000000711 ) ;
#8377=CONICAL_SURFACE ( 'NONE', #1201, 16.50000000000000711, 0.7853981633974447263 ) ;
#8378=VECTOR ( 'NONE', #12027, 1000.000000000000114 ) ;
#8382=CARTESIAN_POINT ( 'NONE',  ( 1.486087262401875941, 13.10364194761998213, 102.0000000000000142 ) ) ;
#8392=AXIS2_PLACEMENT_3D ( 'NONE', #8338, #927, #12245 ) ;
#8393=AXIS2_PLACEMENT_3D ( 'NONE', #5314, #9204, #2881 ) ;
#8397=CARTESIAN_POINT ( 'NONE',  ( 0.000000000000000000, 22.50000000000000000, 101.0000000000000000 ) ) ;
#8400=LINE ( 'NONE', #7409, #2002 ) ;
#8401=DIRECTION ( 'NONE',  ( -0.000000000000000000, -0.000000000000000000, 1.000000000000000000 ) ) ;
#8405=( LENGTH_UNIT ( ) NAMED_UNIT ( * ) SI_UNIT ( .MILLI., .METRE. ) );
#8421=AXIS2_PLACEMENT_3D ( 'NONE', #6755, #4407, #1736 ) ;
#8439=VERTEX_POINT ( 'NONE', #3197 ) ;
#8440=FACE_OUTER_BOUND ( 'NONE', #15710, .T. ) ;
#8442=CONICAL_SURFACE ( 'NONE', #2606, 16.50000000000000711, 0.7853981633974447263 ) ;
#8456=ORIENTED_EDGE ( 'NONE', *, *, #1250, .F. ) ;
#8458=ORIENTED_EDGE ( 'NONE', *, *, #14127, .T. ) ;
#8465=LINE ( 'NONE', #14601, #1570 ) ;
#8467=CARTESIAN_POINT ( 'NONE',  ( 6.251299836021209089, 37.76994598419266680, 102.0000000000000142 ) ) ;
#8468=PLANE ( 'NONE',  #11871 ) ;
#8470=PLANE ( 'NONE',  #2718 ) ;
#8473=VERTEX_POINT ( 'NONE', #4602 ) ;
#8475=ORIENTED_EDGE ( 'NONE', *, *, #5533, .F. ) ;
#8476=EDGE_CURVE ( 'NONE', #7924, #960, #6734, .T. ) ;
#8483=CYLINDRICAL_SURFACE ( 'NONE', #4146, 17.50000000000000000 ) ;
#8495=ORIENTED_EDGE ( 'NONE', *, *, #6633, .F. ) ;
#8501=LINE ( 'NONE', #4865, #4160 ) ;
#8517=ORIENTED_EDGE ( 'NONE', *, *, #5866, .T. ) ;
#8525=VERTEX_POINT ( 'NONE', #7346 ) ;
#8532=DIRECTION ( 'NONE',  ( -1.000000000000000000, 0.000000000000000000, 0.000000000000000000 ) ) ;
#8533=CARTESIAN_POINT ( 'NONE',  ( -9.395693774364753281, 21.00971865127312199, 102.0000000000000142 ) ) ;
#8546=ORIENTED_EDGE ( 'NONE', *, *, #11726, .T. ) ;
#8547=ORIENTED_EDGE ( 'NONE', *, *, #4107, .T. ) ;
#8551=ORIENTED_EDGE ( 'NONE', *, *, #14343, .T. ) ;
#8553=SURFACE_SIDE_STYLE ('',( #13302 ) ) ;
#8557=DIRECTION ( 'NONE',  ( 0.000000000000000000, 0.000000000000000000, -1.000000000000000000 ) ) ;
#8560=DIRECTION ( 'NONE',  ( 1.000000000000000000, 0.000000000000000000, 0.000000000000000000 ) ) ;
#8561=DIRECTION ( 'NONE',  ( -1.224646799147353207E-16, 1.000000000000000000, 0.000000000000000000 ) ) ;
#8563=DIRECTION ( 'NONE',  ( 1.000000000000000000, 0.000000000000000000, 0.000000000000000000 ) ) ;
#8580=DIRECTION ( 'NONE',  ( 0.000000000000000000, 0.000000000000000000, -1.000000000000000000 ) ) ;
#8585=EDGE_CURVE ( 'NONE', #286, #7551, #3344, .T. ) ;
#8590=AXIS2_PLACEMENT_3D ( 'NONE', #8244, #4515, #6095 ) ;
#8592=AXIS2_PLACEMENT_3D ( 'NONE', #3565, #6147, #7469 ) ;
#8593=VERTEX_POINT ( 'NONE', #11086 ) ;
#8601=ORIENTED_EDGE ( 'NONE', *, *, #10664, .F. ) ;
#8603=LINE ( 'NONE', #2292, #11328 ) ;
#8604=ORIENTED_EDGE ( 'NONE', *, *, #16075, .F. ) ;
#8612=LINE ( 'NONE', #7465, #8994 ) ;
#8632=CARTESIAN_POINT ( 'NONE',  ( 0.5000000000000009992, 31.99999999999998579, 101.0000000000000000 ) ) ;
#8636=CARTESIAN_POINT ( 'NONE',  ( -17.11764542475608053, 21.20361710786370324, 101.3333374614808662 ) ) ;
#8639=CARTESIAN_POINT ( 'NONE',  ( -16.48218589020113001, 28.38111794481753236, 101.0000000000000000 ) ) ;
#8641=DIRECTION ( 'NONE',  ( 0.5877852522924688072, 0.8090169943749505599, 0.000000000000000000 ) ) ;
#8644=( GEOMETRIC_REPRESENTATION_CONTEXT ( 3 ) GLOBAL_UNCERTAINTY_ASSIGNED_CONTEXT ( ( #1918 ) ) GLOBAL_UNIT_ASSIGNED_CONTEXT ( ( #12798, #6492, #16463 ) ) REPRESENTATION_CONTEXT ( 'NONE', 'WORKASPACE' ) );
#8647=CARTESIAN_POINT ( 'NONE',  ( 0.000000000000000000, 22.50000000000000000, 102.0000000000000142 ) ) ;
#8651=CARTESIAN_POINT ( 'NONE',  ( 5.179451399591075145, 14.52044592729181538, 101.0000000000000000 ) ) ;
#8656=VECTOR ( 'NONE', #8069, 999.9999999999998863 ) ;
#8661=CARTESIAN_POINT ( 'NONE',  ( -14.90544456622763470, 13.31698729810771376, 102.0000000000000142 ) ) ;
#8664=CARTESIAN_POINT ( 'NONE',  ( 9.151574469205522533, 1.945227203041487218, 101.0000000000000000 ) ) ;
#8666=CARTESIAN_POINT ( 'NONE',  ( -6.725310538855818976, 29.22831317314782851, 102.0000000000000142 ) ) ;
#8672=DIRECTION ( 'NONE',  ( -0.4067366430757887175, -0.9135454576426059736, 0.000000000000000000 ) ) ;
#8713=ORIENTED_EDGE ( 'NONE', *, *, #4643, .F. ) ;
#8716=ORIENTED_EDGE ( 'NONE', *, *, #6509, .T. ) ;
#8726=DIRECTION ( 'NONE',  ( -0.000000000000000000, -0.000000000000000000, -1.000000000000000000 ) ) ;
#8729=CARTESIAN_POINT ( 'NONE',  ( 7.574663982647604321, 38.28367718720770796, 102.0000000000000142 ) ) ;
#8730=EDGE_CURVE ( 'NONE', #7924, #9110, #3590, .T. ) ;
#8736=CARTESIAN_POINT ( 'NONE',  ( -14.32166083077703966, 13.65403499491864459, 101.6666710451724214 ) ) ;
#8738=CIRCLE ( 'NONE', #14313, 6.000000000000001776 ) ;
#8744=EDGE_CURVE ( 'NONE', #404, #7399, #10220, .T. ) ;
#8746=PLANE ( 'NONE',  #15549 ) ;
#8764=ORIENTED_EDGE ( 'NONE', *, *, #5533, .T. ) ;
#8771=CARTESIAN_POINT ( 'NONE',  ( -13.33429048796512717, 33.83343271840278277, 101.0000000000000000 ) ) ;
#8774=CARTESIAN_POINT ( 'NONE',  ( 12.59082374547730332, 33.16401225666611197, 102.0000000000000142 ) ) ;
#8780=DIRECTION ( 'NONE',  ( 1.224646799147353207E-16, -1.000000000000000000, 0.000000000000000000 ) ) ;
#8785=DIRECTION ( 'NONE',  ( -0.5877852522924797984, 0.8090169943749424553, 0.000000000000000000 ) ) ;
#8786=DIRECTION ( 'NONE',  ( -0.000000000000000000, -0.000000000000000000, 1.000000000000000000 ) ) ;
#8792=LINE ( 'NONE', #3898, #13078 ) ;
#8801=CARTESIAN_POINT ( 'NONE',  ( 17.45639740057861644, 21.16801284050037424, 101.0000000000000000 ) ) ;
#8802=CARTESIAN_POINT ( 'NONE',  ( 0.000000000000000000, 0.000000000000000000, 101.0000000000000000 ) ) ;
#8817=VERTEX_POINT ( 'NONE', #3414 ) ;
#8827=CARTESIAN_POINT ( 'NONE',  ( -2.464234863135557063, 13.31155363843772932, 101.0000000000000000 ) ) ;
#8838=AXIS2_PLACEMENT_3D ( 'NONE', #11946, #14352, #544 ) ;
#8843=ORIENTED_EDGE ( 'NONE', *, *, #13016, .T. ) ;
#8853=EDGE_CURVE ( 'NONE', #605, #9440, #7077, .T. ) ;
#8871=AXIS2_PLACEMENT_3D ( 'NONE', #7170, #8561, #10984 ) ;
#8881=VERTEX_POINT ( 'NONE', #13705 ) ;
#8886=LINE ( 'NONE', #13944, #4144 ) ;
#8891=LINE ( 'NONE', #13950, #4971 ) ;
#8892=PLANE ( 'NONE',  #9389 ) ;
#8901=ORIENTED_EDGE ( 'NONE', *, *, #5743, .F. ) ;
#8903=EDGE_LOOP ( 'NONE', ( #8551, #6042, #10575, #14612 ) ) ;
#8904=CARTESIAN_POINT ( 'NONE',  ( 0.000000000000000000, 22.50000000000000000, 101.0000000000000000 ) ) ;
#8925=ORIENTED_EDGE ( 'NONE', *, *, #9653, .F. ) ;
#8930=EDGE_CURVE ( 'NONE', #15550, #8086, #8358, .T. ) ;
#8937=CONICAL_SURFACE ( 'NONE', #14492, 16.50000000000000711, 0.7853981633974447263 ) ;
#8938=VECTOR ( 'NONE', #729, 1000.000000000000000 ) ;
#8946=EDGE_CURVE ( 'NONE', #1083, #9777, #5356, .T. ) ;
#8954=DIRECTION ( 'NONE',  ( 0.1045284632676436315, 0.9945218953682742891, 0.000000000000000000 ) ) ;
#8957=LINE ( 'NONE', #2548, #9983 ) ;
#8959=AXIS2_PLACEMENT_3D ( 'NONE', #996, #8323, #13388 ) ;
#8961=AXIS2_PLACEMENT_3D ( 'NONE', #12712, #2568, #13864 ) ;
#8970=VECTOR ( 'NONE', #889, 1000.000000000000000 ) ;
#8971=ORIENTED_EDGE ( 'NONE', *, *, #3489, .F. ) ;
#8977=CARTESIAN_POINT ( 'NONE',  ( 0.000000000000000000, 22.50000000000000000, 102.0000000000000142 ) ) ;
#8985=CARTESIAN_POINT ( 'NONE',  ( 0.000000000000000000, 22.50000000000000000, 101.0000000000000000 ) ) ;
#8994=VECTOR ( 'NONE', #8786, 1000.000000000000000 ) ;
#9002=DIRECTION ( 'NONE',  ( 0.000000000000000000, -0.000000000000000000, 1.000000000000000000 ) ) ;
#9005=ADVANCED_FACE ( 'NONE', ( #13946 ), #15784, .T. ) ;
#9013=ORIENTED_EDGE ( 'NONE', *, *, #12004, .F. ) ;
#9016=VERTEX_POINT ( 'NONE', #5258 ) ;
#9021=DIRECTION ( 'NONE',  ( 0.000000000000000000, 0.000000000000000000, -1.000000000000000000 ) ) ;
#9023=PLANE ( 'NONE',  #10255 ) ;
#9037=CARTESIAN_POINT ( 'NONE',  ( 14.82166083077715513, 14.52006039870328458, 101.6666710451724214 ) ) ;
#9047=CARTESIAN_POINT ( 'NONE',  ( -9.289494224341229511, 8.863457290943159705, 102.0000000000000142 ) ) ;
#9051=ORIENTED_EDGE ( 'NONE', *, *, #4907, .F. ) ;
#9056=DIRECTION ( 'NONE',  ( -1.000000000000000000, 0.000000000000000000, 0.000000000000000000 ) ) ;
#9057=EDGE_CURVE ( 'NONE', #15672, #9777, #9707, .T. ) ;
#9065=ADVANCED_FACE ( 'NONE', ( #14034 ), #10061, .F. ) ;
#9072=ORIENTED_EDGE ( 'NONE', *, *, #10150, .F. ) ;
#9074=ORIENTED_EDGE ( 'NONE', *, *, #14423, .F. ) ;
#9080=CARTESIAN_POINT ( 'NONE',  ( 0.000000000000000000, 22.50000000000000000, 101.0000000000000000 ) ) ;
#9095=VERTEX_POINT ( 'NONE', #2649 ) ;
#9103=CARTESIAN_POINT ( 'NONE',  ( -12.59082374547745076, 33.16401225666594854, 102.0000000000000142 ) ) ;
#9110=VERTEX_POINT ( 'NONE', #6403 ) ;
#9112=AXIS2_PLACEMENT_3D ( 'NONE', #15796, #574, #14217 ) ;
#9119=CARTESIAN_POINT ( 'NONE',  ( 10.69075041230586365, 8.636095224584757091, 102.0000000000000142 ) ) ;
#9122=CARTESIAN_POINT ( 'NONE',  ( 6.725310538855729270, 29.22831317314791733, 101.0000000000000000 ) ) ;
#9123=VECTOR ( 'NONE', #8401, 1000.000000000000000 ) ;
#9140=FACE_OUTER_BOUND ( 'NONE', #13219, .T. ) ;
#9143=CARTESIAN_POINT ( 'NONE',  ( -10.09851121871618140, 9.451242543235633065, 102.0000000000000142 ) ) ;
#9150=ORIENTED_EDGE ( 'NONE', *, *, #16075, .T. ) ;
#9163=ADVANCED_FACE ( 'NONE', ( #309 ), #15525, .T. ) ;
#9172=CARTESIAN_POINT ( 'NONE',  ( -2.464234863135557063, 13.31155363843772932, 101.0000000000000000 ) ) ;
#9201=CONICAL_SURFACE ( 'NONE', #12106, 16.50000000000000711, 0.7853981633974447263 ) ;
#9204=DIRECTION ( 'NONE',  ( -0.000000000000000000, -0.000000000000000000, -1.000000000000000000 ) ) ;
#9205=CARTESIAN_POINT ( 'NONE',  ( 7.164845293663816506, 37.36320934111687109, 102.0000000000000142 ) ) ;
#9217=CARTESIAN_POINT ( 'NONE',  ( -17.35186893731094671, 20.17349094513186358, 101.0000000000000000 ) ) ;
#9235=CARTESIAN_POINT ( 'NONE',  ( -10.49054022437444900, 8.911660907547297228, 101.3333374614808662 ) ) ;
#9239=DIRECTION ( 'NONE',  ( -0.9135454576426059736, 0.4067366430757887730, 0.000000000000000000 ) ) ;
#9248=EDGE_LOOP ( 'NONE', ( #5179, #14238, #8366, #1389 ) ) ;
#9260=CARTESIAN_POINT ( 'NONE',  ( -1.486087262401750042, 13.10364194761997503, 101.0000000000000000 ) ) ;
#9261=ORIENTED_EDGE ( 'NONE', *, *, #2391, .T. ) ;
#9272=VECTOR ( 'NONE', #14285, 1000.000000000000000 ) ;
#9275=DIRECTION ( 'NONE',  ( 0.000000000000000000, 0.000000000000000000, 1.000000000000000000 ) ) ;
#9277=EDGE_CURVE ( 'NONE', #8192, #11778, #1735, .T. ) ;
#9281=COLOUR_RGB ( '', 0.31764706, 0.68627451, 0.89019608) ;
#9286=DIRECTION ( 'NONE',  ( 0.8660254037844363761, 0.5000000000000041078, 0.000000000000000000 ) ) ;
#9294=AXIS2_PLACEMENT_3D ( 'NONE', #7889, #5259, #15366 ) ;
#9306=DIRECTION ( 'NONE',  ( 1.000000000000000000, 0.000000000000000000, 0.000000000000000000 ) ) ;
#9318=EDGE_CURVE ( 'NONE', #14633, #4499, #5471, .T. ) ;
#9327=ORIENTED_EDGE ( 'NONE', *, *, #13339, .F. ) ;
#9334=DIRECTION ( 'NONE',  ( -0.000000000000000000, 0.000000000000000000, 1.000000000000000000 ) ) ;
#9340=CARTESIAN_POINT ( 'NONE',  ( 12.59082374547730332, 33.16401225666611197, 102.0000000000000142 ) ) ;
#9341=ORIENTED_EDGE ( 'NONE', *, *, #3535, .F. ) ;
#9351=DIRECTION ( 'NONE',  ( 0.8090169943749426773, 0.5877852522924797984, 0.000000000000000000 ) ) ;
#9364=LINE ( 'NONE', #11768, #11552 ) ;
#9369=FACE_OUTER_BOUND ( 'NONE', #15442, .T. ) ;
#9370=EDGE_CURVE ( 'NONE', #1499, #15672, #7512, .T. ) ;
#9378=VERTEX_POINT ( 'NONE', #3557 ) ;
#9379=ORIENTED_EDGE ( 'NONE', *, *, #12255, .T. ) ;
#9387=CARTESIAN_POINT ( 'NONE',  ( 0.000000000000000000, 22.50000000000000000, 101.0000000000000000 ) ) ;
#9389=AXIS2_PLACEMENT_3D ( 'NONE', #10145, #2655, #8641 ) ;
#9401=AXIS2_PLACEMENT_3D ( 'NONE', #1130, #3895, #4996 ) ;
#9418=CARTESIAN_POINT ( 'NONE',  ( 12.83864924538547037, 33.38715533906356114, 101.6666710451724214 ) ) ;
#9422=DIRECTION ( 'NONE',  ( 0.000000000000000000, 0.000000000000000000, 1.000000000000000000 ) ) ;
#9425=ADVANCED_FACE ( 'NONE', ( #5890 ), #12347, .T. ) ;
#9427=DIRECTION ( 'NONE',  ( 1.000000000000000000, 0.000000000000000000, 0.000000000000000000 ) ) ;
#9436=AXIS2_PLACEMENT_3D ( 'NONE', #8802, #11541, #9056 ) ;
#9438=ADVANCED_FACE ( 'NONE', ( #9798 ), #7303, .F. ) ;
#9440=VERTEX_POINT ( 'NONE', #3476 ) ;
#9444=AXIS2_PLACEMENT_3D ( 'NONE', #3691, #925, #7352 ) ;
#9447=EDGE_CURVE ( 'NONE', #14378, #14510, #3302, .T. ) ;
#9463=LINE ( 'NONE', #8212, #2850 ) ;
#9469=AXIS2_PLACEMENT_3D ( 'NONE', #13911, #14247, #9427 ) ;
#9470=AXIS2_PLACEMENT_3D ( 'NONE', #1148, #2729, #7807 ) ;
#9472=LINE ( 'NONE', #8140, #9272 ) ;
#9473=AXIS2_PLACEMENT_3D ( 'NONE', #6678, #4337, #13138 ) ;
#9476=DIRECTION ( 'NONE',  ( 0.1045284632676570929, -0.9945218953682730678, 0.000000000000000000 ) ) ;
#9478=FACE_OUTER_BOUND ( 'NONE', #11128, .T. ) ;
#9484=AXIS2_PLACEMENT_3D ( 'NONE', #5346, #3065, #12973 ) ;
#9488=ORIENTED_EDGE ( 'NONE', *, *, #15187, .T. ) ;
#9494=LINE ( 'NONE', #11898, #8656 ) ;
#9503=DIRECTION ( 'NONE',  ( 0.9510565162951503115, 0.3090169943749573878, 0.000000000000000000 ) ) ;
#9504=EDGE_CURVE ( 'NONE', #12958, #12158, #10492, .T. ) ;
#9510=ORIENTED_EDGE ( 'NONE', *, *, #11413, .F. ) ;
#9526=VERTEX_POINT ( 'NONE', #12028 ) ;
#9528=ORIENTED_EDGE ( 'NONE', *, *, #10122, .T. ) ;
#9529=ORIENTED_EDGE ( 'NONE', *, *, #6958, .F. ) ;
#9546=ORIENTED_EDGE ( 'NONE', *, *, #3052, .F. ) ;
#9565=ORIENTED_EDGE ( 'NONE', *, *, #2391, .F. ) ;
#9568=EDGE_CURVE ( 'NONE', #11934, #13988, #8368, .T. ) ;
#9573=EDGE_CURVE ( 'NONE', #5931, #8153, #5147, .T. ) ;
#9574=FACE_OUTER_BOUND ( 'NONE', #5767, .T. ) ;
#9589=EDGE_LOOP ( 'NONE', ( #11949, #16282, #1310, #778 ) ) ;
#9602=VERTEX_POINT ( 'NONE', #12696 ) ;
#9617=EDGE_LOOP ( 'NONE', ( #4557, #1561, #8475, #15544 ) ) ;
#9623=CARTESIAN_POINT ( 'NONE',  ( 15.84787772126904137, 28.17501872725030054, 101.6666710451724214 ) ) ;
#9628=DIRECTION ( 'NONE',  ( 1.000000000000000000, 0.000000000000000000, 0.000000000000000000 ) ) ;
#9630=DIRECTION ( 'NONE',  ( 0.4067366430758010964, -0.9135454576426004225, 0.000000000000000000 ) ) ;
#9633=FACE_OUTER_BOUND ( 'NONE', #5906, .T. ) ;
#9650=CARTESIAN_POINT ( 'NONE',  ( 16.79799753235259985, 27.43226914341417810, 102.0000000000000142 ) ) ;
#9653=EDGE_CURVE ( 'NONE', #7385, #8473, #10456, .T. ) ;
#9676=CARTESIAN_POINT ( 'NONE',  ( -22.37674264578617311, 24.85189042352198285, 101.0000000000000000 ) ) ;
#9680=EDGE_CURVE ( 'NONE', #3901, #8154, #2546, .T. ) ;
#9691=AXIS2_PLACEMENT_3D ( 'NONE', #10698, #5794, #462 ) ;
#9698=EDGE_CURVE ( 'NONE', #13963, #4275, #1044, .T. ) ;
#9707=CIRCLE ( 'NONE', #398, 16.50000000000000711 ) ;
#9713=FACE_OUTER_BOUND ( 'NONE', #14688, .T. ) ;
#9716=DIRECTION ( 'NONE',  ( -0.9135454576426004225, -0.4067366430758009854, 0.000000000000000000 ) ) ;
#9722=DIRECTION ( 'NONE',  ( -0.9945218953682744001, 0.1045284632676435205, 0.000000000000000000 ) ) ;
#9725=LINE ( 'NONE', #3405, #15185 ) ;
#9727=ORIENTED_EDGE ( 'NONE', *, *, #15135, .T. ) ;
#9730=ORIENTED_EDGE ( 'NONE', *, *, #9870, .T. ) ;
#9736=FACE_OUTER_BOUND ( 'NONE', #9589, .T. ) ;
#9739=VERTEX_POINT ( 'NONE', #9955 ) ;
#9740=LINE ( 'NONE', #15117, #16051 ) ;
#9750=DIRECTION ( 'NONE',  ( -0.3090169943749573878, 0.9510565162951503115, 0.000000000000000000 ) ) ;
#9753=LINE ( 'NONE', #11245, #1485 ) ;
#9755=DIRECTION ( 'NONE',  ( 0.8090169943749426773, 0.5877852522924797984, 0.000000000000000000 ) ) ;
#9756=ORIENTED_EDGE ( 'NONE', *, *, #11915, .F. ) ;
#9761=DIRECTION ( 'NONE',  ( 0.000000000000000000, -0.000000000000000000, -1.000000000000000000 ) ) ;
#9763=AXIS2_PLACEMENT_3D ( 'NONE', #12695, #3884, #14010 ) ;
#9777=VERTEX_POINT ( 'NONE', #9205 ) ;
#9779=EDGE_CURVE ( 'NONE', #404, #10305, #1533, .T. ) ;
#9780=EDGE_CURVE ( 'NONE', #691, #2224, #9364, .T. ) ;
#9781=ORIENTED_EDGE ( 'NONE', *, *, #15187, .F. ) ;
#9782=EDGE_CURVE ( 'NONE', #1083, #1499, #4394, .T. ) ;
#9795=ORIENTED_EDGE ( 'NONE', *, *, #7444, .T. ) ;
#9797=DIRECTION ( 'NONE',  ( -0.000000000000000000, -0.000000000000000000, 1.000000000000000000 ) ) ;
#9798=FACE_OUTER_BOUND ( 'NONE', #16280, .T. ) ;
#9802=DIRECTION ( 'NONE',  ( -0.3090169943749448977, -0.9510565162951543083, 0.000000000000000000 ) ) ;
#9804=CARTESIAN_POINT ( 'NONE',  ( -2.267949192431125027, 22.50000000000000000, 100.0000000000000000 ) ) ;
#9806=DIRECTION ( 'NONE',  ( 0.000000000000000000, 0.000000000000000000, -1.000000000000000000 ) ) ;
#9807=PLANE ( 'NONE',  #7885 ) ;
#9809=ORIENTED_EDGE ( 'NONE', *, *, #9568, .F. ) ;
#9818=ORIENTED_EDGE ( 'NONE', *, *, #5159, .T. ) ;
#9823=LINE ( 'NONE', #3329, #9123 ) ;
#9824=CARTESIAN_POINT ( 'NONE',  ( 5.179451399591075145, 14.52044592729181538, 101.0000000000000000 ) ) ;
#9825=CARTESIAN_POINT ( 'NONE',  ( 0.000000000000000000, 22.50000000000000000, 101.0000000000000000 ) ) ;
#9834=CARTESIAN_POINT ( 'NONE',  ( 0.000000000000000000, 22.50000000000000000, 101.0000000000000000 ) ) ;
#9835=DIRECTION ( 'NONE',  ( -0.000000000000000000, 0.000000000000000000, 1.000000000000000000 ) ) ;
#9844=DIRECTION ( 'NONE',  ( 1.000000000000000000, 0.000000000000000000, 0.000000000000000000 ) ) ;
#9857=ORIENTED_EDGE ( 'NONE', *, *, #1002, .T. ) ;
#9858=CARTESIAN_POINT ( 'NONE',  ( -10.69075041230567891, 8.636095224584611429, 101.0000000000000000 ) ) ;
#9867=EDGE_LOOP ( 'NONE', ( #3861, #9379, #4914, #6896 ) ) ;
#9870=EDGE_CURVE ( 'NONE', #14534, #8275, #1791, .T. ) ;
#9871=EDGE_LOOP ( 'NONE', ( #11806, #10182, #3409, #11247 ) ) ;
#9872=ORIENTED_EDGE ( 'NONE', *, *, #12442, .T. ) ;
#9874=FACE_OUTER_BOUND ( 'NONE', #3368, .T. ) ;
#9876=ADVANCED_FACE ( 'NONE', ( #14092 ), #5315, .F. ) ;
#9887=ORIENTED_EDGE ( 'NONE', *, *, #7951, .T. ) ;
#9890=ORIENTED_EDGE ( 'NONE', *, *, #6374, .F. ) ;
#9891=ORIENTED_EDGE ( 'NONE', *, *, #9504, .T. ) ;
#9898=CARTESIAN_POINT ( 'NONE',  ( -4.320770838041405604, 30.97531352606679178, 102.0000000000000142 ) ) ;
#9899=FACE_OUTER_BOUND ( 'NONE', #15631, .T. ) ;
#9916=CIRCLE ( 'NONE', #13896, 17.50000000000000000 ) ;
#9934=EDGE_LOOP ( 'NONE', ( #77, #2126, #13356, #12955 ) ) ;
#9939=PLANE ( 'NONE',  #16314 ) ;
#9955=CARTESIAN_POINT ( 'NONE',  ( 7.977241335952203194, 17.31698729810786475, 102.0000000000000142 ) ) ;
#9983=VECTOR ( 'NONE', #44, 1000.000000000000000 ) ;
#9985=DIRECTION ( 'NONE',  ( 1.000000000000000000, 0.000000000000000000, 0.000000000000000000 ) ) ;
#9986=CIRCLE ( 'NONE', #12095, 17.50000000000000000 ) ;
#9988=EDGE_CURVE ( 'NONE', #7989, #2880, #14739, .T. ) ;
#9989=LINE ( 'NONE', #6246, #14694 ) ;
#9995=TOROIDAL_SURFACE ( 'NONE', #15563, 7.732050807568878525, 2.000000000000000000 ) ;
#9996=EDGE_LOOP ( 'NONE', ( #8601, #6227, #6103, #10706 ) ) ;
#10005=DIRECTION ( 'NONE',  ( 1.000000000000000000, -2.577303450022684939E-15, 0.000000000000000000 ) ) ;
#10006=EDGE_CURVE ( 'NONE', #1819, #12542, #6107, .T. ) ;
#10024=CONICAL_SURFACE ( 'NONE', #3105, 16.50000000000000711, 0.7853981633974447263 ) ;
#10040=CARTESIAN_POINT ( 'NONE',  ( -0.5000000000000000000, 39.99999999999999289, 102.0000000000000142 ) ) ;
#10043=PLANE ( 'NONE',  #9763 ) ;
#10052=CARTESIAN_POINT ( 'NONE',  ( 9.500222237632415911, 22.00424054664152607, 101.0000000000000000 ) ) ;
#10054=ORIENTED_EDGE ( 'NONE', *, *, #11726, .F. ) ;
#10059=VERTEX_POINT ( 'NONE', #4866 ) ;
#10060=FACE_OUTER_BOUND ( 'NONE', #2809, .T. ) ;
#10061=PLANE ( 'NONE',  #9436 ) ;
#10069=ADVANCED_FACE ( 'NONE', ( #14975 ), #8746, .F. ) ;
#10080=ORIENTED_EDGE ( 'NONE', *, *, #6005, .T. ) ;
#10082=EDGE_CURVE ( 'NONE', #14108, #5931, #9986, .T. ) ;
#10084=DIRECTION ( 'NONE',  ( 0.2079116908177531253, 0.9781476007338069101, 0.000000000000000000 ) ) ;
#10087=DIRECTION ( 'NONE',  ( 0.9510565162951544194, -0.3090169943749448422, 0.000000000000000000 ) ) ;
#10092=VECTOR ( 'NONE', #3667, 1000.000000000000000 ) ;
#10120=ORIENTED_EDGE ( 'NONE', *, *, #10664, .T. ) ;
#10122=EDGE_CURVE ( 'NONE', #6731, #4841, #2422, .T. ) ;
#10125=CARTESIAN_POINT ( 'NONE',  ( -2.267949192431125027, 22.50000000000000000, 102.0000000000000142 ) ) ;
#10142=CARTESIAN_POINT ( 'NONE',  ( 7.977241335952203194, 17.31698729810786475, 101.0000000000000000 ) ) ;
#10144=CARTESIAN_POINT ( 'NONE',  ( 4.127528389677815213, 5.486372832567310454, 101.0000000000000000 ) ) ;
#10145=CARTESIAN_POINT ( 'NONE',  ( -9.881733417930727015, 8.048309972292139847, 101.0000000000000000 ) ) ;
#10150=EDGE_CURVE ( 'NONE', #7907, #7744, #4784, .T. ) ;
#10152=EDGE_CURVE ( 'NONE', #8881, #7781, #4948, .T. ) ;
#10156=ORIENTED_EDGE ( 'NONE', *, *, #14343, .F. ) ;
#10162=EDGE_LOOP ( 'NONE', ( #5206, #15787, #13806, #1826, #12448, #7598, #4479, #14394, #7659, #24, #14784, #9261, #10816, #6653, #2316, #5535, #9488, #15500, #9795, #8716 ) ) ;
#10178=ORIENTED_EDGE ( 'NONE', *, *, #4990, .T. ) ;
#10180=ADVANCED_FACE ( 'NONE', ( #1864 ), #6960, .T. ) ;
#10182=ORIENTED_EDGE ( 'NONE', *, *, #2358, .F. ) ;
#10183=ORIENTED_EDGE ( 'NONE', *, *, #4782, .F. ) ;
#10189=FACE_OUTER_BOUND ( 'NONE', #1291, .T. ) ;
#10194=EDGE_CURVE ( 'NONE', #12675, #2743, #5483, .T. ) ;
#10208=EDGE_CURVE ( 'NONE', #15183, #6731, #6508, .T. ) ;
#10220=CIRCLE ( 'NONE', #11023, 17.50000000000000000 ) ;
#10240=VECTOR ( 'NONE', #11178, 1000.000000000000000 ) ;
#10244=VECTOR ( 'NONE', #3506, 1000.000000000000000 ) ;
#10255=AXIS2_PLACEMENT_3D ( 'NONE', #7769, #195, #7611 ) ;
#10268=AXIS2_PLACEMENT_3D ( 'NONE', #1266, #6357, #3852 ) ;
#10271=AXIS2_PLACEMENT_3D ( 'NONE', #4827, #14935, #11217 ) ;
#10285=ADVANCED_FACE ( 'NONE', ( #3844 ), #14136, .T. ) ;
#10289=ORIENTED_EDGE ( 'NONE', *, *, #4782, .T. ) ;
#10305=VERTEX_POINT ( 'NONE', #174 ) ;
#10310=DIRECTION ( 'NONE',  ( 1.000000000000000000, 0.000000000000000000, 0.000000000000000000 ) ) ;
#10312=CARTESIAN_POINT ( 'NONE',  ( -16.68146630878711534, 20.24395310072295828, 101.6666710451724214 ) ) ;
#10315=DIRECTION ( 'NONE',  ( -0.9945218953682730678, -0.1045284632676570929, 0.000000000000000000 ) ) ;
#10319=CARTESIAN_POINT ( 'NONE',  ( -6.251299836021416922, 37.76994598419257443, 102.0000000000000142 ) ) ;
#10320=VERTEX_POINT ( 'NONE', #7826 ) ;
#10335=FACE_OUTER_BOUND ( 'NONE', #11707, .T. ) ;
#10343=ORIENTED_EDGE ( 'NONE', *, *, #15667, .F. ) ;
#10348=DIRECTION ( 'NONE',  ( 0.9781476007338069101, -0.2079116908177532641, 0.000000000000000000 ) ) ;
#10363=ORIENTED_EDGE ( 'NONE', *, *, #10776, .F. ) ;
#10377=B_SPLINE_CURVE_WITH_KNOTS ( 'NONE', 3,
 ( #5472, #15600, #13342, #1945 ),
 .UNSPECIFIED., .F., .F.,
 ( 4, 4 ),
 ( 2.829004760683457170E-07, 0.001414802801989366787 ),
 .UNSPECIFIED. ) ;
#10379=ADVANCED_FACE ( 'NONE', ( #5754, #6851 ), #5433, .T. ) ;
#10381=ORIENTED_EDGE ( 'NONE', *, *, #6633, .T. ) ;
#10386=EDGE_LOOP ( 'NONE', ( #9891, #818, #3578, #5385 ) ) ;
#10389=DIRECTION ( 'NONE',  ( 1.000000000000000000, 0.000000000000000000, 0.000000000000000000 ) ) ;
#10405=VERTEX_POINT ( 'NONE', #10659 ) ;
#10407=DIRECTION ( 'NONE',  ( 1.000000000000000000, 0.000000000000000000, 0.000000000000000000 ) ) ;
#10412=CARTESIAN_POINT ( 'NONE',  ( -16.48898053797772789, 28.38332565970911148, 101.0000000000000000 ) ) ;
#10413=CARTESIAN_POINT ( 'NONE',  ( -15.40544456622763470, 14.18301270189214947, 101.0000000000000000 ) ) ;
#10416=B_SPLINE_CURVE_WITH_KNOTS ( 'NONE', 3,
 ( #2663, #322, #4076, #10319 ),
 .UNSPECIFIED., .F., .F.,
 ( 4, 4 ),
 ( 2.829004760709176796E-07, 0.001414802801989367437 ),
 .UNSPECIFIED. ) ;
#10445=VECTOR ( 'NONE', #5606, 1000.000000000000000 ) ;
#10456=B_SPLINE_CURVE_WITH_KNOTS ( 'NONE', 3,
 ( #1123, #3647, #7463, #6304 ),
 .UNSPECIFIED., .F., .F.,
 ( 4, 4 ),
 ( 2.829004760671193191E-07, 0.001414802801989368305 ),
 .UNSPECIFIED. ) ;
#10458=LINE ( 'NONE', #6395, #7774 ) ;
#10461=VERTEX_POINT ( 'NONE', #3169 ) ;
#10463=ORIENTED_EDGE ( 'NONE', *, *, #11329, .T. ) ;
#10465=CARTESIAN_POINT ( 'NONE',  ( 15.53071739328000334, 28.07196708982297295, 102.0000000000000142 ) ) ;
#10481=AXIS2_PLACEMENT_3D ( 'NONE', #193, #15487, #7931 ) ;
#10486=EDGE_CURVE ( 'NONE', #13541, #12113, #13066, .T. ) ;
#10492=B_SPLINE_CURVE_WITH_KNOTS ( 'NONE', 3,
 ( #4645, #15861, #9623, #13524 ),
 .UNSPECIFIED., .F., .F.,
 ( 4, 4 ),
 ( 2.829004760679149478E-07, 0.001414802801989366787 ),
 .UNSPECIFIED. ) ;
#10495=AXIS2_PLACEMENT_3D ( 'NONE', #1948, #3207, #15847 ) ;
#10496=CARTESIAN_POINT ( 'NONE',  ( 0.000000000000000000, 22.50000000000000000, 101.0000000000000000 ) ) ;
#10500=CARTESIAN_POINT ( 'NONE',  ( 2.464234863135679188, 13.31155363843775064, 101.0000000000000000 ) ) ;
#10511=ORIENTED_EDGE ( 'NONE', *, *, #1765, .F. ) ;
#10522=AXIS2_PLACEMENT_3D ( 'NONE', #2977, #11954, #6976 ) ;
#10524=CARTESIAN_POINT ( 'NONE',  ( 0.000000000000000000, 22.50000000000000000, 102.0000000000000142 ) ) ;
#10533=VECTOR ( 'NONE', #2596, 1000.000000000000000 ) ;
#10534=VECTOR ( 'NONE', #14893, 1000.000000000000227 ) ;
#10540=EDGE_CURVE ( 'NONE', #15183, #13963, #4521, .T. ) ;
#10547=CIRCLE ( 'NONE', #10268, 17.50000000000000000 ) ;
#10550=CIRCLE ( 'NONE', #12668, 16.50000000000000711 ) ;
#10557=ORIENTED_EDGE ( 'NONE', *, *, #4292, .T. ) ;
#10559=DIRECTION ( 'NONE',  ( 0.7431448254773955764, -0.6691306063588567943, 0.000000000000000000 ) ) ;
#10567=CARTESIAN_POINT ( 'NONE',  ( 0.000000000000000000, 22.50000000000000000, 101.0000000000000000 ) ) ;
#10575=ORIENTED_EDGE ( 'NONE', *, *, #12401, .F. ) ;
#10586=PLANE ( 'NONE',  #1487 ) ;
#10590=EDGE_CURVE ( 'NONE', #14668, #12113, #8400, .T. ) ;
#10596=ADVANCED_FACE ( 'NONE', ( #4845 ), #8483, .T. ) ;
#10599=ORIENTED_EDGE ( 'NONE', *, *, #12600, .F. ) ;
#10602=ADVANCED_FACE ( 'NONE', ( #12226 ), #4928, .T. ) ;
#10631=EDGE_LOOP ( 'NONE', ( #6446, #4215, #14206, #6798 ) ) ;
#10659=CARTESIAN_POINT ( 'NONE',  ( 3.407225380398686276, 31.38205016914263723, 101.0000000000000000 ) ) ;
#10664=EDGE_CURVE ( 'NONE', #10059, #12675, #2280, .T. ) ;
#10665=LINE ( 'NONE', #8243, #2481 ) ;
#10671=LINE ( 'NONE', #9260, #2733 ) ;
#10693=VECTOR ( 'NONE', #7714, 1000.000000000000000 ) ;
#10698=CARTESIAN_POINT ( 'NONE',  ( 0.000000000000000000, 22.50000000000000000, 102.0000000000000142 ) ) ;
#10706=ORIENTED_EDGE ( 'NONE', *, *, #112, .F. ) ;
#10710=EDGE_CURVE ( 'NONE', #7385, #14428, #12916, .T. ) ;
#10715=DIRECTION ( 'NONE',  ( 0.000000000000000000, 0.000000000000000000, -1.000000000000000000 ) ) ;
#10721=CARTESIAN_POINT ( 'NONE',  ( 21.39877161664097471, 15.54711762656373786, 101.0000000000000000 ) ) ;
#10736=LINE ( 'NONE', #4427, #14666 ) ;
#10740=CARTESIAN_POINT ( 'NONE',  ( 0.000000000000000000, 22.50000000000000000, 102.0000000000000142 ) ) ;
#10752=FACE_BOUND ( 'NONE', #16305, .T. ) ;
#10755=B_SPLINE_CURVE_WITH_KNOTS ( 'NONE', 3,
 ( #15429, #4049, #14959, #3747 ),
 .UNSPECIFIED., .F., .F.,
 ( 4, 4 ),
 ( 0.01140363079879802566, 0.01281815069648909247 ),
 .UNSPECIFIED. ) ;
#10770=ORIENTED_EDGE ( 'NONE', *, *, #5523, .T. ) ;
#10771=ORIENTED_EDGE ( 'NONE', *, *, #15459, .F. ) ;
#10775=VECTOR ( 'NONE', #3439, 1000.000000000000000 ) ;
#10776=EDGE_CURVE ( 'NONE', #860, #1083, #7078, .T. ) ;
#10784=EDGE_CURVE ( 'NONE', #8473, #7372, #1219, .T. ) ;
#10785=EDGE_CURVE ( 'NONE', #9110, #16246, #5170, .T. ) ;
#10789=AXIS2_PLACEMENT_3D ( 'NONE', #6770, #13147, #12905 ) ;
#10790=VECTOR ( 'NONE', #8315, 1000.000000000000000 ) ;
#10792=AXIS2_PLACEMENT_3D ( 'NONE', #16460, #6241, #2485 ) ;
#10794=EDGE_CURVE ( 'NONE', #14575, #11298, #8891, .T. ) ;
#10807=DIRECTION ( 'NONE',  ( 1.000000000000000000, 1.685159948091755373E-14, 0.000000000000000000 ) ) ;
#10808=DIRECTION ( 'NONE',  ( 0.000000000000000000, 0.000000000000000000, -1.000000000000000000 ) ) ;
#10816=ORIENTED_EDGE ( 'NONE', *, *, #1369, .T. ) ;
#10862=EDGE_CURVE ( 'NONE', #11303, #8275, #3911, .T. ) ;
#10871=ORIENTED_EDGE ( 'NONE', *, *, #3871, .F. ) ;
#10876=DIRECTION ( 'NONE',  ( 1.000000000000000000, 0.000000000000000000, 0.000000000000000000 ) ) ;
#10877=CARTESIAN_POINT ( 'NONE',  ( 17.45639740057861644, 21.16801284050037424, 101.0000000000000000 ) ) ;
#10891=ORIENTED_EDGE ( 'NONE', *, *, #15569, .F. ) ;
#10903=EDGE_CURVE ( 'NONE', #6731, #4275, #8603, .T. ) ;
#10907=PLANE ( 'NONE',  #13202 ) ;
#10911=VERTEX_POINT ( 'NONE', #874 ) ;
#10914=ORIENTED_EDGE ( 'NONE', *, *, #4192, .T. ) ;
#10918=EDGE_CURVE ( 'NONE', #13582, #2974, #7536, .T. ) ;
#10920=CARTESIAN_POINT ( 'NONE',  ( -9.189545401991425777, 24.96013318841439599, 101.0000000000000000 ) ) ;
#10944=DIRECTION ( 'NONE',  ( -1.000000000000000000, 0.000000000000000000, 0.000000000000000000 ) ) ;
#10953=CARTESIAN_POINT ( 'NONE',  ( 12.66515988160610107, 34.57657754388035443, 101.0000000000000000 ) ) ;
#10962=VECTOR ( 'NONE', #14233, 1000.000000000000000 ) ;
#10968=ORIENTED_EDGE ( 'NONE', *, *, #760, .F. ) ;
#10972=DIRECTION ( 'NONE',  ( 0.000000000000000000, 0.000000000000000000, -1.000000000000000000 ) ) ;
#10973=AXIS2_PLACEMENT_3D ( 'NONE', #15529, #313, #6904 ) ;
#10974=ORIENTED_EDGE ( 'NONE', *, *, #10710, .F. ) ;
#10976=SURFACE_STYLE_USAGE ( .BOTH. , #8553 ) ;
#10984=DIRECTION ( 'NONE',  ( -1.000000000000000000, 0.000000000000000000, 0.000000000000000000 ) ) ;
#11018=ORIENTED_EDGE ( 'NONE', *, *, #9447, .T. ) ;
#11023=AXIS2_PLACEMENT_3D ( 'NONE', #8904, #6421, #10407 ) ;
#11033=EDGE_LOOP ( 'NONE', ( #8232, #12217, #9051, #5270 ) ) ;
#11035=ORIENTED_EDGE ( 'NONE', *, *, #5567, .F. ) ;
#11048=CIRCLE ( 'NONE', #9470, 7.732050807568878525 ) ;
#11051=VECTOR ( 'NONE', #14809, 1000.000000000000114 ) ;
#11053=DIRECTION ( 'NONE',  ( -0.3090169943749448422, -0.9510565162951544194, 0.000000000000000000 ) ) ;
#11071=FACE_OUTER_BOUND ( 'NONE', #3517, .T. ) ;
#11073=DIRECTION ( 'NONE',  ( 0.000000000000000000, 0.000000000000000000, 1.000000000000000000 ) ) ;
#11074=CARTESIAN_POINT ( 'NONE',  ( -8.880528407616480990, 25.91118970470954963, 101.0000000000000000 ) ) ;
#11086=CARTESIAN_POINT ( 'NONE',  ( -8.477241335952138357, 18.18301270189218855, 102.0000000000000142 ) ) ;
#11088=FACE_OUTER_BOUND ( 'NONE', #4941, .T. ) ;
#11092=CARTESIAN_POINT ( 'NONE',  ( 9.395693774364776374, 21.00971865127324634, 101.0000000000000000 ) ) ;
#11128=EDGE_LOOP ( 'NONE', ( #977, #6658, #4636, #10054 ) ) ;
#11129=ORIENTED_EDGE ( 'NONE', *, *, #4751, .T. ) ;
#11130=ORIENTED_EDGE ( 'NONE', *, *, #7339, .F. ) ;
#11131=DIRECTION ( 'NONE',  ( 0.7431448254773955764, -0.6691306063588567943, 0.000000000000000000 ) ) ;
#11143=CARTESIAN_POINT ( 'NONE',  ( -16.79799753235266735, 27.43226914341395783, 101.0000000000000000 ) ) ;
#11146=ORIENTED_EDGE ( 'NONE', *, *, #760, .T. ) ;
#11150=VECTOR ( 'NONE', #2152, 1000.000000000000000 ) ;
#11153=VERTEX_POINT ( 'NONE', #6868 ) ;
#11156=DIRECTION ( 'NONE',  ( 0.000000000000000000, 0.000000000000000000, -1.000000000000000000 ) ) ;
#11157=DIRECTION ( 'NONE',  ( -1.000000000000000000, 0.000000000000000000, 0.000000000000000000 ) ) ;
#11160=DIRECTION ( 'NONE',  ( 0.4999999999999920064, 0.8660254037844432595, 0.000000000000000000 ) ) ;
#11169=DIRECTION ( 'NONE',  ( 1.000000000000000000, -1.784287003861858895E-15, 0.000000000000000000 ) ) ;
#11173=EDGE_LOOP ( 'NONE', ( #9565, #13186, #15108, #5129 ) ) ;
#11178=DIRECTION ( 'NONE',  ( -0.2079116908177665590, 0.9781476007338041345, 0.000000000000000000 ) ) ;
#11208=ORIENTED_EDGE ( 'NONE', *, *, #2254, .T. ) ;
#11217=DIRECTION ( 'NONE',  ( 1.000000000000000000, 0.000000000000000000, 0.000000000000000000 ) ) ;
#11218=CARTESIAN_POINT ( 'NONE',  ( -17.50000000000000000, 22.50000000000000000, 102.0000000000000142 ) ) ;
#11225=ADVANCED_FACE ( 'NONE', ( #10752, #8256 ), #13160, .T. ) ;
#11226=ADVANCED_FACE ( 'NONE', ( #14559 ), #13320, .T. ) ;
#11231=CARTESIAN_POINT ( 'NONE',  ( -7.977241335952133916, 17.31698729810774751, 101.0000000000000000 ) ) ;
#11233=DIRECTION ( 'NONE',  ( 1.000000000000000000, 0.000000000000000000, 0.000000000000000000 ) ) ;
#11238=FACE_OUTER_BOUND ( 'NONE', #7496, .T. ) ;
#11245=CARTESIAN_POINT ( 'NONE',  ( 13.33959974903368995, 33.83821319854147447, 101.0000000000000000 ) ) ;
#11247=ORIENTED_EDGE ( 'NONE', *, *, #7662, .T. ) ;
#11252=EDGE_CURVE ( 'NONE', #2031, #12133, #1005, .T. ) ;
#11255=DIRECTION ( 'NONE',  ( 0.8090169943749504489, -0.5877852522924689183, 0.000000000000000000 ) ) ;
#11260=DIRECTION ( 'NONE',  ( 1.000000000000000000, 0.000000000000000000, -0.000000000000000000 ) ) ;
#11272=VECTOR ( 'NONE', #9630, 1000.000000000000114 ) ;
#11273=CARTESIAN_POINT ( 'NONE',  ( 8.477241335952196977, 18.18301270189230578, 101.0000000000000000 ) ) ;
#11274=CARTESIAN_POINT ( 'NONE',  ( 0.000000000000000000, 22.50000000000000000, 102.0000000000000142 ) ) ;
#11284=EDGE_CURVE ( 'NONE', #14151, #7383, #13563, .T. ) ;
#11298=VERTEX_POINT ( 'NONE', #14804 ) ;
#11303=VERTEX_POINT ( 'NONE', #12493 ) ;
#11310=CARTESIAN_POINT ( 'NONE',  ( -17.44929222242214095, 21.16875962481669760, 101.0000000000000000 ) ) ;
#11327=CIRCLE ( 'NONE', #4159, 17.50000000000000000 ) ;
#11328=VECTOR ( 'NONE', #2375, 1000.000000000000000 ) ;
#11329=EDGE_CURVE ( 'NONE', #8439, #6384, #2169, .T. ) ;
#11343=AXIS2_PLACEMENT_3D ( 'NONE', #8632, #2229, #12472 ) ;
#11349=ADVANCED_FACE ( 'NONE', ( #11088 ), #3098, .T. ) ;
#11350=ORIENTED_EDGE ( 'NONE', *, *, #3232, .F. ) ;
#11353=ORIENTED_EDGE ( 'NONE', *, *, #8853, .T. ) ;
#11370=CARTESIAN_POINT ( 'NONE',  ( 9.395693774364776374, 21.00971865127324634, 102.0000000000000142 ) ) ;
#11389=ORIENTED_EDGE ( 'NONE', *, *, #9698, .T. ) ;
#11391=DIRECTION ( 'NONE',  ( 0.000000000000000000, 0.000000000000000000, -1.000000000000000000 ) ) ;
#11395=DIRECTION ( 'NONE',  ( 0.000000000000000000, 0.000000000000000000, -1.000000000000000000 ) ) ;
#11409=DIRECTION ( 'NONE',  ( 1.000000000000000000, 0.000000000000000000, 0.000000000000000000 ) ) ;
#11413=EDGE_CURVE ( 'NONE', #2743, #12041, #2590, .T. ) ;
#11420=PLANE ( 'NONE',  #14243 ) ;
#11435=CARTESIAN_POINT ( 'NONE',  ( 9.395693774364776374, 21.00971865127324634, 102.0000000000000142 ) ) ;
#11447=VERTEX_POINT ( 'NONE', #12810 ) ;
#11448=LINE ( 'NONE', #11370, #7595 ) ;
#11449=DIRECTION ( 'NONE',  ( -0.9135454576426004225, -0.4067366430758009854, 0.000000000000000000 ) ) ;
#11456=DIRECTION ( 'NONE',  ( 0.1045284632676572456, -0.9945218953682730678, -0.000000000000000000 ) ) ;
#11457=ORIENTED_EDGE ( 'NONE', *, *, #10862, .T. ) ;
#11459=ORIENTED_EDGE ( 'NONE', *, *, #9573, .T. ) ;
#11471=FILL_AREA_STYLE ('',( #11548 ) ) ;
#11476=LINE ( 'NONE', #7815, #12121 ) ;
#11477=ORIENTED_EDGE ( 'NONE', *, *, #8203, .F. ) ;
#11484=AXIS2_PLACEMENT_3D ( 'NONE', #9217, #11456, #301 ) ;
#11485=ORIENTED_EDGE ( 'NONE', *, *, #6509, .F. ) ;
#11490=CARTESIAN_POINT ( 'NONE',  ( 17.35186893731097868, 20.17349094513210161, 102.0000000000000142 ) ) ;
#11495=CARTESIAN_POINT ( 'NONE',  ( -9.395693774364753281, 21.00971865127312199, 101.0000000000000000 ) ) ;
#11524=DIRECTION ( 'NONE',  ( -0.7071067811865451302, 0.000000000000000000, -0.7071067811865500152 ) ) ;
#11537=CARTESIAN_POINT ( 'NONE',  ( -0.4999999999999998890, 38.99242250247064590, 102.0000000000000142 ) ) ;
#11541=DIRECTION ( 'NONE',  ( -0.000000000000000000, 0.000000000000000000, -1.000000000000000000 ) ) ;
#11548=FILL_AREA_STYLE_COLOUR ( '', #4135 ) ;
#11551=CARTESIAN_POINT ( 'NONE',  ( -16.79120288457607657, 27.43006142852237517, 101.0000000000000000 ) ) ;
#11552=VECTOR ( 'NONE', #11690, 1000.000000000000000 ) ;
#11560=DIRECTION ( 'NONE',  ( 1.000000000000000000, 0.000000000000000000, 0.000000000000000000 ) ) ;
#11573=CARTESIAN_POINT ( 'NONE',  ( 0.000000000000000000, 22.50000000000000000, 80.00000000000000000 ) ) ;
#11575=CARTESIAN_POINT ( 'NONE',  ( 17.50000000000000000, 22.50000000000000355, 101.0000000000000000 ) ) ;
#11576=CIRCLE ( 'NONE', #16097, 17.50000000000000000 ) ;
#11589=EDGE_CURVE ( 'NONE', #3858, #1326, #12735, .T. ) ;
#11597=CARTESIAN_POINT ( 'NONE',  ( -3.009228475883398257, 5.937825933686429636, 101.6666710451724214 ) ) ;
#11607=AXIS2_PLACEMENT_3D ( 'NONE', #8985, #2660, #4168 ) ;
#11613=ORIENTED_EDGE ( 'NONE', *, *, #8476, .T. ) ;
#11626=DIRECTION ( 'NONE',  ( 0.000000000000000000, 0.000000000000000000, -1.000000000000000000 ) ) ;
#11655=DIRECTION ( 'NONE',  ( 1.000000000000000000, 0.000000000000000000, 0.000000000000000000 ) ) ;
#11656=LINE ( 'NONE', #7910, #1932 ) ;
#11658=DIRECTION ( 'NONE',  ( -0.9135454576426005335, -0.4067366430758011520, 0.000000000000000000 ) ) ;
#11682=EDGE_CURVE ( 'NONE', #2031, #13278, #10550, .T. ) ;
#11690=DIRECTION ( 'NONE',  ( -0.000000000000000000, -0.000000000000000000, 1.000000000000000000 ) ) ;
#11695=CARTESIAN_POINT ( 'NONE',  ( 7.977241335952203194, 17.31698729810786475, 101.0000000000000000 ) ) ;
#11699=EDGE_CURVE ( 'NONE', #2224, #12941, #14376, .T. ) ;
#11701=DIRECTION ( 'NONE',  ( 1.000000000000000000, 0.000000000000000000, 0.000000000000000000 ) ) ;
#11706=FACE_OUTER_BOUND ( 'NONE', #9871, .T. ) ;
#11707=EDGE_LOOP ( 'NONE', ( #12999, #11748, #6882, #1702 ) ) ;
#11726=EDGE_CURVE ( 'NONE', #1499, #1769, #7987, .T. ) ;
#11730=EDGE_LOOP ( 'NONE', ( #13058, #189, #1685, #6398 ) ) ;
#11735=DIRECTION ( 'NONE',  ( 0.000000000000000000, 0.000000000000000000, 1.000000000000000000 ) ) ;
#11739=CARTESIAN_POINT ( 'NONE',  ( 7.977241335952203194, 17.31698729810786475, 102.0000000000000142 ) ) ;
#11744=EDGE_CURVE ( 'NONE', #7461, #9095, #6919, .T. ) ;
#11747=EDGE_CURVE ( 'NONE', #4841, #6384, #15791, .T. ) ;
#11748=ORIENTED_EDGE ( 'NONE', *, *, #3464, .F. ) ;
#11751=DIRECTION ( 'NONE',  ( -0.2079116908177532641, -0.9781476007338069101, 0.000000000000000000 ) ) ;
#11758=CIRCLE ( 'NONE', #8838, 17.50000000000000000 ) ;
#11768=CARTESIAN_POINT ( 'NONE',  ( 9.189545401991395579, 24.96013318841451678, 101.0000000000000000 ) ) ;
#11769=CARTESIAN_POINT ( 'NONE',  ( 4.320770838041294581, 30.97531352606685218, 101.0000000000000000 ) ) ;
#11778=VERTEX_POINT ( 'NONE', #569 ) ;
#11784=ORIENTED_EDGE ( 'NONE', *, *, #6634, .T. ) ;
#11788=AXIS2_PLACEMENT_3D ( 'NONE', #4567, #10808, #14857 ) ;
#11793=LINE ( 'NONE', #15619, #13512 ) ;
#11795=EDGE_CURVE ( 'NONE', #15183, #13541, #13982, .T. ) ;
#11796=FACE_OUTER_BOUND ( 'NONE', #9867, .T. ) ;
#11799=CARTESIAN_POINT ( 'NONE',  ( -2.464234863135557063, 13.31155363843772932, 101.0000000000000000 ) ) ;
#11802=CIRCLE ( 'NONE', #10481, 16.50000000000000711 ) ;
#11805=ORIENTED_EDGE ( 'NONE', *, *, #9780, .F. ) ;
#11806=ORIENTED_EDGE ( 'NONE', *, *, #15452, .F. ) ;
#11810=ORIENTED_EDGE ( 'NONE', *, *, #3877, .T. ) ;
#11811=PLANE ( 'NONE',  #13171 ) ;
#11812=DIRECTION ( 'NONE',  ( 0.7431448254773955764, -0.6691306063588567943, 0.000000000000000000 ) ) ;
#11813=DIRECTION ( 'NONE',  ( 1.000000000000000000, -7.137148015447435579E-15, 0.000000000000000000 ) ) ;
#11819=DIRECTION ( 'NONE',  ( 0.4999999999999919509, 0.8660254037844432595, 0.000000000000000000 ) ) ;
#11830=CARTESIAN_POINT ( 'NONE',  ( -17.34476375915448187, 20.17423772944842142, 101.0000000000000000 ) ) ;
#11840=ADVANCED_FACE ( 'NONE', ( #5748 ), #5429, .F. ) ;
#11846=CIRCLE ( 'NONE', #13960, 16.50000000000000711 ) ;
#11851=AXIS2_PLACEMENT_3D ( 'NONE', #13548, #11156, #11233 ) ;
#11852=VECTOR ( 'NONE', #3518, 999.9999999999998863 ) ;
#11854=ORIENTED_EDGE ( 'NONE', *, *, #10590, .T. ) ;
#11861=AXIS2_PLACEMENT_3D ( 'NONE', #9676, #8580, #7362 ) ;
#11863=VECTOR ( 'NONE', #2779, 1000.000000000000000 ) ;
#11871=AXIS2_PLACEMENT_3D ( 'NONE', #16026, #11963, #5652 ) ;
#11873=PLANE ( 'NONE',  #13995 ) ;
#11894=DIRECTION ( 'NONE',  ( -1.000000000000000000, -1.224646799147353207E-16, 0.000000000000000000 ) ) ;
#11896=EDGE_LOOP ( 'NONE', ( #10599, #9072, #16128, #12757 ) ) ;
#11897=AXIS2_PLACEMENT_3D ( 'NONE', #7470, #1470, #13935 ) ;
#11898=CARTESIAN_POINT ( 'NONE',  ( -9.500222237632405253, 22.00424054664139817, 102.0000000000000142 ) ) ;
#11900=LINE ( 'NONE', #15640, #12286 ) ;
#11905=CARTESIAN_POINT ( 'NONE',  ( 14.90544456622775904, 13.31698729810792692, 102.0000000000000142 ) ) ;
#11908=CARTESIAN_POINT ( 'NONE',  ( 6.658212670116058440, 38.68388717334331517, 101.0000000000000000 ) ) ;
#11912=CARTESIAN_POINT ( 'NONE',  ( 3.149380788944009968, 5.278461141749541063, 102.0000000000000142 ) ) ;
#11915=EDGE_CURVE ( 'NONE', #14633, #8275, #742, .T. ) ;
#11929=ADVANCED_FACE ( 'NONE', ( #9736 ), #7161, .T. ) ;
#11934=VERTEX_POINT ( 'NONE', #16037 ) ;
#11946=CARTESIAN_POINT ( 'NONE',  ( 0.000000000000000000, 22.50000000000000000, 101.0000000000000000 ) ) ;
#11949=ORIENTED_EDGE ( 'NONE', *, *, #12382, .F. ) ;
#11954=DIRECTION ( 'NONE',  ( 0.000000000000000000, 0.000000000000000000, 1.000000000000000000 ) ) ;
#11963=DIRECTION ( 'NONE',  ( -0.6691306063588673414, 0.7431448254773861395, 0.000000000000000000 ) ) ;
#11972=CARTESIAN_POINT ( 'NONE',  ( -9.189545401991425777, 24.96013318841439599, 101.0000000000000000 ) ) ;
#11976=CARTESIAN_POINT ( 'NONE',  ( -6.661118525005218949, 38.69041383028340420, 101.0000000000000000 ) ) ;
#11988=EDGE_LOOP ( 'NONE', ( #1564, #10463, #13374, #717 ) ) ;
#11991=VERTEX_POINT ( 'NONE', #7076 ) ;
#11997=ADVANCED_FACE ( 'NONE', ( #5008 ), #15851, .T. ) ;
#12001=CARTESIAN_POINT ( 'NONE',  ( 9.395693774364776374, 21.00971865127324634, 101.0000000000000000 ) ) ;
#12004=EDGE_CURVE ( 'NONE', #7385, #14575, #1141, .T. ) ;
#12022=ORIENTED_EDGE ( 'NONE', *, *, #1798, .T. ) ;
#12023=CIRCLE ( 'NONE', #345, 17.50000000000000000 ) ;
#12027=DIRECTION ( 'NONE',  ( 0.4067366430758010964, -0.9135454576426004225, 0.000000000000000000 ) ) ;
#12028=CARTESIAN_POINT ( 'NONE',  ( 2.267949192431125027, 22.50000000000000000, 102.0000000000000142 ) ) ;
#12034=VECTOR ( 'NONE', #9802, 1000.000000000000114 ) ;
#12035=CARTESIAN_POINT ( 'NONE',  ( 4.320770838041294581, 30.97531352606685218, 101.0000000000000000 ) ) ;
#12040=DIRECTION ( 'NONE',  ( 0.000000000000000000, -0.000000000000000000, -1.000000000000000000 ) ) ;
#12041=VERTEX_POINT ( 'NONE', #2648 ) ;
#12052=CARTESIAN_POINT ( 'NONE',  ( -4.126043002969710827, 5.493361027597350343, 101.0000000000000000 ) ) ;
#12054=CARTESIAN_POINT ( 'NONE',  ( -1.486087262401750042, 13.10364194761997503, 101.0000000000000000 ) ) ;
#12061=FACE_OUTER_BOUND ( 'NONE', #16204, .T. ) ;
#12082=AXIS2_PLACEMENT_3D ( 'NONE', #8213, #4064, #8046 ) ;
#12092=ORIENTED_EDGE ( 'NONE', *, *, #3820, .T. ) ;
#12095=AXIS2_PLACEMENT_3D ( 'NONE', #14894, #12322, #10005 ) ;
#12100=EDGE_CURVE ( 'NONE', #691, #7234, #8886, .T. ) ;
#12101=VECTOR ( 'NONE', #9351, 999.9999999999998863 ) ;
#12106=AXIS2_PLACEMENT_3D ( 'NONE', #16231, #3690, #13809 ) ;
#12108=AXIS2_PLACEMENT_3D ( 'NONE', #64, #11395, #14115 ) ;
#12111=ORIENTED_EDGE ( 'NONE', *, *, #6195, .T. ) ;
#12112=ADVANCED_FACE ( 'NONE', ( #10060 ), #6483, .F. ) ;
#12113=VERTEX_POINT ( 'NONE', #3985 ) ;
#12116=CARTESIAN_POINT ( 'NONE',  ( -3.407225380398804404, 31.38205016914259105, 102.0000000000000142 ) ) ;
#12119=AXIS2_PLACEMENT_3D ( 'NONE', #13816, #15395, #15068 ) ;
#12121=VECTOR ( 'NONE', #9239, 1000.000000000000000 ) ;
#12126=DIRECTION ( 'NONE',  ( -0.4067366430757887175, -0.9135454576426059736, 0.000000000000000000 ) ) ;
#12127=LINE ( 'NONE', #888, #2039 ) ;
#12133=VERTEX_POINT ( 'NONE', #3739 ) ;
#12135=ORIENTED_EDGE ( 'NONE', *, *, #1527, .T. ) ;
#12141=ORIENTED_EDGE ( 'NONE', *, *, #9698, .F. ) ;
#12143=FACE_OUTER_BOUND ( 'NONE', #6848, .T. ) ;
#12147=CARTESIAN_POINT ( 'NONE',  ( 7.394441145214595501, 28.48516834767053751, 102.0000000000000142 ) ) ;
#12148=CARTESIAN_POINT ( 'NONE',  ( 0.000000000000000000, 22.50000000000000000, 101.0000000000000000 ) ) ;
#12152=PLANE ( 'NONE',  #15848 ) ;
#12158=VERTEX_POINT ( 'NONE', #10465 ) ;
#12160=CARTESIAN_POINT ( 'NONE',  ( 0.000000000000000000, 22.50000000000000000, 102.0000000000000142 ) ) ;
#12167=CARTESIAN_POINT ( 'NONE',  ( 8.477241335952196977, 18.18301270189230578, 102.0000000000000142 ) ) ;
#12168=B_SPLINE_CURVE_WITH_KNOTS ( 'NONE', 3,
 ( #15161, #6532, #11597, #3787 ),
 .UNSPECIFIED., .F., .F.,
 ( 4, 4 ),
 ( 2.829004760677457000E-07, 0.001414802801989367004 ),
 .UNSPECIFIED. ) ;
#12174=ADVANCED_BREP_SHAPE_REPRESENTATION ( '', ( #3320, #15812 ), #16077 ) ;
#12176=ORIENTED_EDGE ( 'NONE', *, *, #6070, .T. ) ;
#12185=LINE ( 'NONE', #13669, #13143 ) ;
#12192=ORIENTED_EDGE ( 'NONE', *, *, #11747, .T. ) ;
#12201=CARTESIAN_POINT ( 'NONE',  ( -14.03285685708567065, 13.82077604687239258, 102.0000000000000142 ) ) ;
#12204=LINE ( 'NONE', #5894, #8052 ) ;
#12210=CARTESIAN_POINT ( 'NONE',  ( 17.44929222242216227, 21.16875962481693207, 101.0000000000000000 ) ) ;
#12212=ADVANCED_FACE ( 'NONE', ( #14193 ), #11873, .T. ) ;
#12214=EDGE_LOOP ( 'NONE', ( #3073, #3199, #7686, #15920 ) ) ;
#12217=ORIENTED_EDGE ( 'NONE', *, *, #10150, .T. ) ;
#12218=ORIENTED_EDGE ( 'NONE', *, *, #2468, .T. ) ;
#12224=PLANE ( 'NONE',  #16443 ) ;
#12226=FACE_OUTER_BOUND ( 'NONE', #1622, .T. ) ;
#12241=CARTESIAN_POINT ( 'NONE',  ( -16.79799753235266735, 27.43226914341395783, 102.0000000000000142 ) ) ;
#12243=PLANE ( 'NONE',  #3356 ) ;
#12245=DIRECTION ( 'NONE',  ( 1.000000000000000000, 0.000000000000000000, 0.000000000000000000 ) ) ;
#12255=EDGE_CURVE ( 'NONE', #589, #562, #387, .T. ) ;
#12258=ORIENTED_EDGE ( 'NONE', *, *, #11744, .F. ) ;
#12273=ORIENTED_EDGE ( 'NONE', *, *, #14711, .T. ) ;
#12275=ORIENTED_EDGE ( 'NONE', *, *, #11915, .T. ) ;
#12276=CARTESIAN_POINT ( 'NONE',  ( -7.574663982647817484, 38.28367718720760138, 101.0000000000000000 ) ) ;
#12285=DIRECTION ( 'NONE',  ( -1.000000000000000000, -1.224646799147353207E-16, 0.000000000000000000 ) ) ;
#12286=VECTOR ( 'NONE', #2926, 1000.000000000000227 ) ;
#12293=ORIENTED_EDGE ( 'NONE', *, *, #1527, .F. ) ;
#12297=CIRCLE ( 'NONE', #5154, 17.50000000000000000 ) ;
#12300=PRESENTATION_STYLE_ASSIGNMENT (( #10976 ) ) ;
#12309=CARTESIAN_POINT ( 'NONE',  ( 9.189545401991395579, 24.96013318841451678, 101.0000000000000000 ) ) ;
#12314=CIRCLE ( 'NONE', #11788, 17.50000000000000000 ) ;
#12315=CARTESIAN_POINT ( 'NONE',  ( -16.48218589020113001, 28.38111794481753236, 101.0000000000000000 ) ) ;
#12318=EDGE_LOOP ( 'NONE', ( #5913, #5351, #2068, #13860 ) ) ;
#12319=DIRECTION ( 'NONE',  ( 0.9510565162951544194, -0.3090169943749448422, 0.000000000000000000 ) ) ;
#12321=CARTESIAN_POINT ( 'NONE',  ( 1.486087262401875941, 13.10364194761998213, 102.0000000000000142 ) ) ;
#12322=DIRECTION ( 'NONE',  ( 0.000000000000000000, 0.000000000000000000, -1.000000000000000000 ) ) ;
#12325=CARTESIAN_POINT ( 'NONE',  ( 0.000000000000000000, 22.50000000000000000, 101.0000000000000000 ) ) ;
#12337=EDGE_LOOP ( 'NONE', ( #7048, #9781, #14925, #15840 ) ) ;
#12347=TOROIDAL_SURFACE ( 'NONE', #4946, 2.267949192431125027, 2.000000000000000000 ) ;
#12359=STYLED_ITEM ( 'NONE', ( #6166 ), #12174 ) ;
#12364=AXIS2_PLACEMENT_3D ( 'NONE', #2947, #446, #1779 ) ;
#12377=DIRECTION ( 'NONE',  ( 0.9510565162951544194, -0.3090169943749448422, 0.000000000000000000 ) ) ;
#12382=EDGE_CURVE ( 'NONE', #1101, #2974, #9463, .T. ) ;
#12387=VECTOR ( 'NONE', #342, 1000.000000000000000 ) ;
#12394=ORIENTED_EDGE ( 'NONE', *, *, #4622, .T. ) ;
#12401=EDGE_CURVE ( 'NONE', #793, #8154, #4644, .T. ) ;
#12405=VECTOR ( 'NONE', #13213, 1000.000000000000000 ) ;
#12408=FACE_OUTER_BOUND ( 'NONE', #3488, .T. ) ;
#12411=ORIENTED_EDGE ( 'NONE', *, *, #16217, .F. ) ;
#12417=CIRCLE ( 'NONE', #8959, 17.50000000000000000 ) ;
#12418=CARTESIAN_POINT ( 'NONE',  ( 14.89925740754320493, 13.32055945583997314, 101.0000000000000000 ) ) ;
#12442=EDGE_CURVE ( 'NONE', #7423, #793, #5805, .T. ) ;
#12448=ORIENTED_EDGE ( 'NONE', *, *, #8744, .T. ) ;
#12452=CARTESIAN_POINT ( 'NONE',  ( -16.48898053797772789, 28.38332565970911148, 102.0000000000000142 ) ) ;
#12454=LINE ( 'NONE', #12698, #15621 ) ;
#12459=CARTESIAN_POINT ( 'NONE',  ( 15.40544456622774661, 14.18301270189236973, 102.0000000000000142 ) ) ;
#12460=AXIS2_PLACEMENT_3D ( 'NONE', #1239, #12638, #9985 ) ;
#12469=ORIENTED_EDGE ( 'NONE', *, *, #13474, .F. ) ;
#12472=DIRECTION ( 'NONE',  ( 0.000000000000000000, -0.000000000000000000, 1.000000000000000000 ) ) ;
#12485=PLANE ( 'NONE',  #3917 ) ;
#12490=ORIENTED_EDGE ( 'NONE', *, *, #15170, .T. ) ;
#12493=CARTESIAN_POINT ( 'NONE',  ( -5.988468393965924008, 15.10823117958422301, 102.0000000000000142 ) ) ;
#12507=ADVANCED_FACE ( 'NONE', ( #9874 ), #14926, .F. ) ;
#12511=ORIENTED_EDGE ( 'NONE', *, *, #399, .F. ) ;
#12532=CARTESIAN_POINT ( 'NONE',  ( 22.37674264578614114, 24.85189042352228483, 101.0000000000000000 ) ) ;
#12539=ORIENTED_EDGE ( 'NONE', *, *, #3871, .T. ) ;
#12542=VERTEX_POINT ( 'NONE', #1208 ) ;
#12555=LINE ( 'NONE', #16382, #6552 ) ;
#12556=EDGE_CURVE ( 'NONE', #3156, #14378, #3265, .T. ) ;
#12559=DIRECTION ( 'NONE',  ( -0.4067366430757887175, -0.9135454576426059736, 0.000000000000000000 ) ) ;
#12562=CARTESIAN_POINT ( 'NONE',  ( -14.61046079763414518, 13.48729625631173867, 101.3333374614808662 ) ) ;
#12565=AXIS2_PLACEMENT_3D ( 'NONE', #14390, #15650, #8082 ) ;
#12600=EDGE_CURVE ( 'NONE', #7744, #11298, #11448, .T. ) ;
#12609=DIRECTION ( 'NONE',  ( 0.8660254037844362651, 0.5000000000000041078, 0.000000000000000000 ) ) ;
#12617=CARTESIAN_POINT ( 'NONE',  ( 14.89925740754320493, 13.32055945583997314, 101.0000000000000000 ) ) ;
#12622=AXIS2_PLACEMENT_3D ( 'NONE', #6899, #14431, #10389 ) ;
#12626=ORIENTED_EDGE ( 'NONE', *, *, #3585, .F. ) ;
#12630=DIRECTION ( 'NONE',  ( -0.9945218953682744001, 0.1045284632676435205, 0.000000000000000000 ) ) ;
#12638=DIRECTION ( 'NONE',  ( 0.000000000000000000, 0.000000000000000000, 1.000000000000000000 ) ) ;
#12639=AXIS2_PLACEMENT_3D ( 'NONE', #13469, #7243, #13791 ) ;
#12642=SURFACE_STYLE_USAGE ( .BOTH. , #154 ) ;
#12649=CARTESIAN_POINT ( 'NONE',  ( -14.89925740754307881, 13.32055945583976353, 101.0000000000000000 ) ) ;
#12666=DIRECTION ( 'NONE',  ( 0.000000000000000000, 0.000000000000000000, 1.000000000000000000 ) ) ;
#12668=AXIS2_PLACEMENT_3D ( 'NONE', #1412, #5031, #11560 ) ;
#12675=VERTEX_POINT ( 'NONE', #15254 ) ;
#12677=AXIS2_PLACEMENT_3D ( 'NONE', #836, #16144, #8563 ) ;
#12678=ORIENTED_EDGE ( 'NONE', *, *, #5523, .F. ) ;
#12695=CARTESIAN_POINT ( 'NONE',  ( -8.880528407616480990, 25.91118970470954963, 101.0000000000000000 ) ) ;
#12696=CARTESIAN_POINT ( 'NONE',  ( 0.5000000000000001110, 38.99242250247064590, 102.0000000000000142 ) ) ;
#12697=CARTESIAN_POINT ( 'NONE',  ( -17.50000000000000000, 22.50000000000000000, 101.0000000000000000 ) ) ;
#12698=CARTESIAN_POINT ( 'NONE',  ( -3.149380788943775933, 5.278461141749506425, 102.0000000000000142 ) ) ;
#12704=CARTESIAN_POINT ( 'NONE',  ( -14.53285685708567421, 14.68680145065682474, 102.0000000000000142 ) ) ;
#12712=CARTESIAN_POINT ( 'NONE',  ( 16.72075857324139747, 7.444561356925718520, 101.0000000000000000 ) ) ;
#12713=CARTESIAN_POINT ( 'NONE',  ( 7.571758127758665857, 38.27715053026751946, 101.0000000000000000 ) ) ;
#12714=ADVANCED_FACE ( 'NONE', ( #2459 ), #10043, .T. ) ;
#12719=FACE_OUTER_BOUND ( 'NONE', #11033, .T. ) ;
#12723=EDGE_CURVE ( 'NONE', #8086, #566, #7785, .T. ) ;
#12735=LINE ( 'NONE', #1331, #15036 ) ;
#12739=DIRECTION ( 'NONE',  ( 0.8090169943749425663, 0.5877852522924799095, 0.000000000000000000 ) ) ;
#12740=CARTESIAN_POINT ( 'NONE',  ( 7.394441145214595501, 28.48516834767053751, 101.0000000000000000 ) ) ;
#12742=LINE ( 'NONE', #11490, #10533 ) ;
#12757=ORIENTED_EDGE ( 'NONE', *, *, #10794, .T. ) ;
#12772=ORIENTED_EDGE ( 'NONE', *, *, #9504, .F. ) ;
#12776=CARTESIAN_POINT ( 'NONE',  ( 0.000000000000000000, 22.50000000000000000, 102.0000000000000142 ) ) ;
#12779=CARTESIAN_POINT ( 'NONE',  ( -12.66515988160626982, 34.57657754388018390, 101.0000000000000000 ) ) ;
#12788=ORIENTED_EDGE ( 'NONE', *, *, #2598, .T. ) ;
#12789=ORIENTED_EDGE ( 'NONE', *, *, #10540, .T. ) ;
#12798=( LENGTH_UNIT ( ) NAMED_UNIT ( * ) SI_UNIT ( .MILLI., .METRE. ) );
#12799=CARTESIAN_POINT ( 'NONE',  ( 10.49054022437463018, 8.911660907547437560, 101.3333374614808662 ) ) ;
#12804=ADVANCED_FACE ( 'NONE', ( #12855 ), #7344, .T. ) ;
#12810=CARTESIAN_POINT ( 'NONE',  ( 5.988468393966018155, 15.10823117958429584, 101.0000000000000000 ) ) ;
#12815=DIRECTION ( 'NONE',  ( -0.5877852522924797984, 0.8090169943749424553, 0.000000000000000000 ) ) ;
#12830=ORIENTED_EDGE ( 'NONE', *, *, #15742, .F. ) ;
#12834=ORIENTED_EDGE ( 'NONE', *, *, #10208, .T. ) ;
#12854=ORIENTED_EDGE ( 'NONE', *, *, #9782, .F. ) ;
#12855=FACE_OUTER_BOUND ( 'NONE', #12214, .T. ) ;
#12864=FACE_OUTER_BOUND ( 'NONE', #5741, .T. ) ;
#12866=ORIENTED_EDGE ( 'NONE', *, *, #13116, .T. ) ;
#12883=PLANE ( 'NONE',  #15498 ) ;
#12894=AXIS2_PLACEMENT_3D ( 'NONE', #6900, #1726, #10876 ) ;
#12895=CARTESIAN_POINT ( 'NONE',  ( 0.5000000000000000000, 39.99999999999999289, 101.0000000000000000 ) ) ;
#12901=ADVANCED_FACE ( 'NONE', ( #289 ), #367, .T. ) ;
#12905=DIRECTION ( 'NONE',  ( 0.000000000000000000, 0.000000000000000000, -1.000000000000000000 ) ) ;
#12916=CIRCLE ( 'NONE', #10792, 17.50000000000000000 ) ;
#12939=VECTOR ( 'NONE', #2706, 999.9999999999998863 ) ;
#12941=VERTEX_POINT ( 'NONE', #16311 ) ;
#12946=CARTESIAN_POINT ( 'NONE',  ( -15.11046079763414696, 14.35332166009617261, 101.3333374614808662 ) ) ;
#12955=ORIENTED_EDGE ( 'NONE', *, *, #12100, .F. ) ;
#12957=AXIS2_PLACEMENT_3D ( 'NONE', #10877, #14598, #5892 ) ;
#12958=VERTEX_POINT ( 'NONE', #4947 ) ;
#12960=ORIENTED_EDGE ( 'NONE', *, *, #1873, .T. ) ;
#12961=ORIENTED_EDGE ( 'NONE', *, *, #915, .T. ) ;
#12971=DIRECTION ( 'NONE',  ( 0.7431448254773955764, -0.6691306063588567943, 0.000000000000000000 ) ) ;
#12973=DIRECTION ( 'NONE',  ( 1.000000000000000000, 0.000000000000000000, 0.000000000000000000 ) ) ;
#12976=EDGE_CURVE ( 'NONE', #4332, #11447, #13566, .T. ) ;
#12989=CARTESIAN_POINT ( 'NONE',  ( -9.500222237632405253, 22.00424054664139817, 101.0000000000000000 ) ) ;
#12999=ORIENTED_EDGE ( 'NONE', *, *, #10006, .F. ) ;
#13001=ORIENTED_EDGE ( 'NONE', *, *, #800, .T. ) ;
#13004=AXIS2_PLACEMENT_3D ( 'NONE', #8977, #5167, #10310 ) ;
#13005=CARTESIAN_POINT ( 'NONE',  ( 9.395693774364776374, 21.00971865127324634, 101.0000000000000000 ) ) ;
#13016=EDGE_CURVE ( 'NONE', #7399, #13988, #7253, .T. ) ;
#13018=ORIENTED_EDGE ( 'NONE', *, *, #13590, .F. ) ;
#13027=CARTESIAN_POINT ( 'NONE',  ( -6.725310538855818976, 29.22831317314782851, 101.0000000000000000 ) ) ;
#13028=ADVANCED_FACE ( 'NONE', ( #6180 ), #9201, .T. ) ;
#13031=DIRECTION ( 'NONE',  ( -0.000000000000000000, -0.000000000000000000, 1.000000000000000000 ) ) ;
#13034=VERTEX_POINT ( 'NONE', #12321 ) ;
#13047=CARTESIAN_POINT ( 'NONE',  ( -19.48557158514997312, 33.74999999999982236, 101.0000000000000000 ) ) ;
#13055=DIRECTION ( 'NONE',  ( 0.9945218953682730678, 0.1045284632676572317, 0.000000000000000000 ) ) ;
#13058=ORIENTED_EDGE ( 'NONE', *, *, #13116, .F. ) ;
#13063=ORIENTED_EDGE ( 'NONE', *, *, #8930, .F. ) ;
#13064=EDGE_CURVE ( 'NONE', #14671, #8593, #8501, .T. ) ;
#13066=LINE ( 'NONE', #13142, #13680 ) ;
#13073=CARTESIAN_POINT ( 'NONE',  ( -8.477241335952138357, 18.18301270189218855, 101.0000000000000000 ) ) ;
#13077=ORIENTED_EDGE ( 'NONE', *, *, #6067, .T. ) ;
#13078=VECTOR ( 'NONE', #4142, 999.9999999999998863 ) ;
#13095=ADVANCED_FACE ( 'NONE', ( #2093 ), #12243, .F. ) ;
#13102=CARTESIAN_POINT ( 'NONE',  ( -5.179451399590974781, 14.52044592729175321, 101.0000000000000000 ) ) ;
#13111=EDGE_LOOP ( 'NONE', ( #12834, #15597, #12141, #15324 ) ) ;
#13116=EDGE_CURVE ( 'NONE', #14108, #7047, #5109, .T. ) ;
#13126=CARTESIAN_POINT ( 'NONE',  ( -7.394441145214675437, 28.48516834767043093, 101.0000000000000000 ) ) ;
#13136=EDGE_LOOP ( 'NONE', ( #13263, #9818, #2856, #9341 ) ) ;
#13138=DIRECTION ( 'NONE',  ( 1.000000000000000000, 0.000000000000000000, 0.000000000000000000 ) ) ;
#13142=CARTESIAN_POINT ( 'NONE',  ( -13.33959974903384627, 33.83821319854129683, 101.0000000000000000 ) ) ;
#13143=VECTOR ( 'NONE', #8357, 1000.000000000000000 ) ;
#13147=DIRECTION ( 'NONE',  ( 0.000000000000000000, -1.000000000000000000, 0.000000000000000000 ) ) ;
#13160=PLANE ( 'NONE',  #13436 ) ;
#13170=VECTOR ( 'NONE', #3127, 1000.000000000000000 ) ;
#13171=AXIS2_PLACEMENT_3D ( 'NONE', #11976, #3083, #8160 ) ;
#13172=FACE_OUTER_BOUND ( 'NONE', #13136, .T. ) ;
#13173=AXIS2_PLACEMENT_3D ( 'NONE', #9080, #5358, #11655 ) ;
#13182=AXIS2_PLACEMENT_3D ( 'NONE', #1593, #11735, #337 ) ;
#13186=ORIENTED_EDGE ( 'NONE', *, *, #13339, .T. ) ;
#13195=VECTOR ( 'NONE', #13299, 1000.000000000000000 ) ;
#13202=AXIS2_PLACEMENT_3D ( 'NONE', #7006, #7335, #4433 ) ;
#13213=DIRECTION ( 'NONE',  ( -0.7431448254773861395, -0.6691306063588672304, 0.000000000000000000 ) ) ;
#13219=EDGE_LOOP ( 'NONE', ( #11035, #7642, #719, #14860 ) ) ;
#13224=CARTESIAN_POINT ( 'NONE',  ( 12.67046914267482016, 34.58135802401886139, 101.0000000000000000 ) ) ;
#13233=LINE ( 'NONE', #16215, #479 ) ;
#13251=FACE_OUTER_BOUND ( 'NONE', #11896, .T. ) ;
#13259=TOROIDAL_SURFACE ( 'NONE', #3971, 7.732050807568878525, 2.000000000000000000 ) ;
#13263=ORIENTED_EDGE ( 'NONE', *, *, #14177, .T. ) ;
#13264=CARTESIAN_POINT ( 'NONE',  ( 7.977241335952203194, 17.31698729810786475, 101.0000000000000000 ) ) ;
#13269=PLANE ( 'NONE',  #13421 ) ;
#13278=VERTEX_POINT ( 'NONE', #1827 ) ;
#13293=EDGE_CURVE ( 'NONE', #7383, #4055, #9494, .T. ) ;
#13299=DIRECTION ( 'NONE',  ( -0.2079116908177665590, 0.9781476007338041345, 0.000000000000000000 ) ) ;
#13302=SURFACE_STYLE_FILL_AREA ( #5832 ) ;
#13307=DIRECTION ( 'NONE',  ( -0.9510565162951503115, -0.3090169943749574988, 0.000000000000000000 ) ) ;
#13308=ADVANCED_FACE ( 'NONE', ( #9574 ), #11811, .T. ) ;
#13312=LINE ( 'NONE', #16050, #6856 ) ;
#13315=LINE ( 'NONE', #3340, #15479 ) ;
#13317=ORIENTED_EDGE ( 'NONE', *, *, #2263, .F. ) ;
#13320=PLANE ( 'NONE',  #6288 ) ;
#13334=ORIENTED_EDGE ( 'NONE', *, *, #5685, .T. ) ;
#13339=EDGE_CURVE ( 'NONE', #3858, #4499, #5868, .T. ) ;
#13340=VERTEX_POINT ( 'NONE', #5667 ) ;
#13341=AXIS2_PLACEMENT_3D ( 'NONE', #11143, #11053, #12377 ) ;
#13342=CARTESIAN_POINT ( 'NONE',  ( 3.987376076617427767, 6.145737624504234553, 101.6666710451724214 ) ) ;
#13346=PRODUCT_CONTEXT ( 'NONE', #15337, 'mechanical' ) ;
#13356=ORIENTED_EDGE ( 'NONE', *, *, #16286, .T. ) ;
#13360=CARTESIAN_POINT ( 'NONE',  ( -6.251299836021416922, 37.76994598419257443, 102.0000000000000142 ) ) ;
#13361=CARTESIAN_POINT ( 'NONE',  ( 15.40544456622774661, 14.18301270189236973, 101.0000000000000000 ) ) ;
#13367=CARTESIAN_POINT ( 'NONE',  ( 2.939893647802748866, 6.264020653511243708, 102.0000000000000142 ) ) ;
#13370=DIRECTION ( 'NONE',  ( 1.000000000000000000, 0.000000000000000000, 0.000000000000000000 ) ) ;
#13373=ORIENTED_EDGE ( 'NONE', *, *, #14892, .F. ) ;
#13374=ORIENTED_EDGE ( 'NONE', *, *, #11747, .F. ) ;
#13375=ORIENTED_EDGE ( 'NONE', *, *, #8730, .F. ) ;
#13379=ORIENTED_EDGE ( 'NONE', *, *, #11795, .T. ) ;
#13388=DIRECTION ( 'NONE',  ( 1.000000000000000000, 2.141144404634230516E-14, 0.000000000000000000 ) ) ;
#13393=SHAPE_REPRESENTATION ( 'Speed Control Knob & Dial', ( #15812 ), #16077 ) ;
#13416=EDGE_CURVE ( 'NONE', #3156, #14668, #3001, .T. ) ;
#13418=VECTOR ( 'NONE', #13769, 1000.000000000000114 ) ;
#13421=AXIS2_PLACEMENT_3D ( 'NONE', #13027, #1795, #5712 ) ;
#13423=FACE_OUTER_BOUND ( 'NONE', #694, .T. ) ;
#13434=AXIS2_PLACEMENT_3D ( 'NONE', #9825, #3505, #4674 ) ;
#13435=ORIENTED_EDGE ( 'NONE', *, *, #10194, .T. ) ;
#13436=AXIS2_PLACEMENT_3D ( 'NONE', #1770, #9422, #3103 ) ;
#13438=ORIENTED_EDGE ( 'NONE', *, *, #13416, .T. ) ;
#13449=ADVANCED_FACE ( 'NONE', ( #5519 ), #15638, .F. ) ;
#13455=CARTESIAN_POINT ( 'NONE',  ( 6.725310538855729270, 29.22831317314791733, 101.0000000000000000 ) ) ;
#13457=ORIENTED_EDGE ( 'NONE', *, *, #7051, .T. ) ;
#13461=ORIENTED_EDGE ( 'NONE', *, *, #9870, .F. ) ;
#13467=DIRECTION ( 'NONE',  ( 0.000000000000000000, 0.000000000000000000, -1.000000000000000000 ) ) ;
#13469=CARTESIAN_POINT ( 'NONE',  ( -5.988468393965924008, 15.10823117958422301, 101.0000000000000000 ) ) ;
#13474=EDGE_CURVE ( 'NONE', #1819, #11153, #3880, .T. ) ;
#13477=FACE_OUTER_BOUND ( 'NONE', #1161, .T. ) ;
#13491=DIRECTION ( 'NONE',  ( 1.000000000000000000, 0.000000000000000000, 0.000000000000000000 ) ) ;
#13502=AXIS2_PLACEMENT_3D ( 'NONE', #13047, #10715, #5649 ) ;
#13512=VECTOR ( 'NONE', #1573, 1000.000000000000000 ) ;
#13522=ORIENTED_EDGE ( 'NONE', *, *, #800, .F. ) ;
#13524=CARTESIAN_POINT ( 'NONE',  ( 15.53071739328000334, 28.07196708982297295, 102.0000000000000142 ) ) ;
#13528=CIRCLE ( 'NONE', #3716, 17.50000000000000000 ) ;
#13536=DIRECTION ( 'NONE',  ( 0.9781476007338042455, 0.2079116908177664758, 0.000000000000000000 ) ) ;
#13537=ORIENTED_EDGE ( 'NONE', *, *, #10486, .T. ) ;
#13541=VERTEX_POINT ( 'NONE', #16136 ) ;
#13548=CARTESIAN_POINT ( 'NONE',  ( 0.000000000000000000, 22.50000000000000000, 101.0000000000000000 ) ) ;
#13551=CARTESIAN_POINT ( 'NONE',  ( 13.33429048796497085, 33.83343271840296751, 101.0000000000000000 ) ) ;
#13563=LINE ( 'NONE', #3688, #5501 ) ;
#13566=LINE ( 'NONE', #14718, #10534 ) ;
#13582=VERTEX_POINT ( 'NONE', #6406 ) ;
#13588=ADVANCED_FACE ( 'NONE', ( #12719 ), #148, .T. ) ;
#13590=EDGE_CURVE ( 'NONE', #2880, #7989, #11048, .T. ) ;
#13597=ORIENTED_EDGE ( 'NONE', *, *, #9779, .T. ) ;
#13624=DIRECTION ( 'NONE',  ( 0.000000000000000000, 0.000000000000000000, -1.000000000000000000 ) ) ;
#13628=DIRECTION ( 'NONE',  ( -0.9510565162951503115, -0.3090169943749574988, 0.000000000000000000 ) ) ;
#13629=FACE_OUTER_BOUND ( 'NONE', #1057, .T. ) ;
#13630=EDGE_CURVE ( 'NONE', #8086, #4820, #6855, .T. ) ;
#13639=ORIENTED_EDGE ( 'NONE', *, *, #5945, .F. ) ;
#13644=CARTESIAN_POINT ( 'NONE',  ( 14.03285685708579145, 13.82077604687259154, 102.0000000000000142 ) ) ;
#13667=DIRECTION ( 'NONE',  ( 0.8090169943749505599, -0.5877852522924688072, -0.000000000000000000 ) ) ;
#13669=CARTESIAN_POINT ( 'NONE',  ( 16.48898053797764973, 28.38332565970932819, 102.0000000000000142 ) ) ;
#13670=AXIS2_PLACEMENT_3D ( 'NONE', #212, #7867, #14414 ) ;
#13680=VECTOR ( 'NONE', #11812, 1000.000000000000000 ) ;
#13681=ORIENTED_EDGE ( 'NONE', *, *, #12976, .F. ) ;
#13695=PLANE ( 'NONE',  #13341 ) ;
#13700=EDGE_LOOP ( 'NONE', ( #6176, #3782, #5405, #1085 ) ) ;
#13704=DIRECTION ( 'NONE',  ( 0.5877852522924688072, 0.8090169943749505599, 0.000000000000000000 ) ) ;
#13705=CARTESIAN_POINT ( 'NONE',  ( 7.977241335952203194, 17.31698729810786475, 101.0000000000000000 ) ) ;
#13709=CARTESIAN_POINT ( 'NONE',  ( -16.45433951800529826, 21.27333336793995144, 102.0000000000000142 ) ) ;
#13732=EDGE_CURVE ( 'NONE', #6085, #8525, #557, .T. ) ;
#13734=CARTESIAN_POINT ( 'NONE',  ( -8.880528407616480990, 25.91118970470954963, 101.0000000000000000 ) ) ;
#13735=DIRECTION ( 'NONE',  ( -0.6691306063588569053, -0.7431448254773954654, 0.000000000000000000 ) ) ;
#13746=CIRCLE ( 'NONE', #11897, 2.000000000000000000 ) ;
#13749=ORIENTED_EDGE ( 'NONE', *, *, #10082, .F. ) ;
#13751=DIRECTION ( 'NONE',  ( -0.3090169943749573878, 0.9510565162951503115, 0.000000000000000000 ) ) ;
#13766=EDGE_CURVE ( 'NONE', #12958, #13340, #3639, .T. ) ;
#13769=DIRECTION ( 'NONE',  ( 0.1045284632676436315, 0.9945218953682742891, 0.000000000000000000 ) ) ;
#13773=DIRECTION ( 'NONE',  ( 0.000000000000000000, 0.000000000000000000, -1.000000000000000000 ) ) ;
#13782=ORIENTED_EDGE ( 'NONE', *, *, #13016, .F. ) ;
#13791=DIRECTION ( 'NONE',  ( 0.8090169943749505599, -0.5877852522924689183, 0.000000000000000000 ) ) ;
#13794=DIRECTION ( 'NONE',  ( -0.5877852522924797984, 0.8090169943749424553, 0.000000000000000000 ) ) ;
#13796=DIRECTION ( 'NONE',  ( 0.5877852522924688072, 0.8090169943749505599, 0.000000000000000000 ) ) ;
#13801=EDGE_CURVE ( 'NONE', #10305, #6366, #7147, .T. ) ;
#13803=CARTESIAN_POINT ( 'NONE',  ( 16.79799753235259985, 27.43226914341417810, 101.0000000000000000 ) ) ;
#13806=ORIENTED_EDGE ( 'NONE', *, *, #10710, .T. ) ;
#13809=DIRECTION ( 'NONE',  ( -1.000000000000000000, 0.000000000000000000, 0.000000000000000000 ) ) ;
#13816=CARTESIAN_POINT ( 'NONE',  ( -4.678013043399745108, 44.50832101651058537, 101.0000000000000000 ) ) ;
#13823=ORIENTED_EDGE ( 'NONE', *, *, #11682, .T. ) ;
#13824=EDGE_CURVE ( 'NONE', #12158, #1479, #7096, .T. ) ;
#13831=DIRECTION ( 'NONE',  ( 0.000000000000000000, 0.000000000000000000, -1.000000000000000000 ) ) ;
#13833=CARTESIAN_POINT ( 'NONE',  ( -12.83864924538561780, 33.38715533906339061, 101.6666710451724214 ) ) ;
#13835=EDGE_CURVE ( 'NONE', #4080, #8192, #6828, .T. ) ;
#13847=CARTESIAN_POINT ( 'NONE',  ( -16.50000000000000711, 22.50000000000000000, 102.0000000000000142 ) ) ;
#13856=FACE_OUTER_BOUND ( 'NONE', #11988, .T. ) ;
#13860=ORIENTED_EDGE ( 'NONE', *, *, #3362, .T. ) ;
#13861=EDGE_LOOP ( 'NONE', ( #8713, #5723, #14952, #744 ) ) ;
#13864=DIRECTION ( 'NONE',  ( -0.6691306063588569053, -0.7431448254773954654, 0.000000000000000000 ) ) ;
#13882=ORIENTED_EDGE ( 'NONE', *, *, #8946, .F. ) ;
#13896=AXIS2_PLACEMENT_3D ( 'NONE', #10496, #4184, #11813 ) ;
#13908=CIRCLE ( 'NONE', #7546, 17.50000000000000000 ) ;
#13911=CARTESIAN_POINT ( 'NONE',  ( 0.000000000000000000, 22.50000000000000000, 102.0000000000000142 ) ) ;
#13919=CARTESIAN_POINT ( 'NONE',  ( 0.000000000000000000, 22.50000000000000000, 102.0000000000000142 ) ) ;
#13929=DIRECTION ( 'NONE',  ( -1.000000000000000000, 0.000000000000000000, 0.000000000000000000 ) ) ;
#13935=DIRECTION ( 'NONE',  ( -1.000000000000000000, 0.000000000000000000, 0.000000000000000000 ) ) ;
#13938=VECTOR ( 'NONE', #11131, 1000.000000000000000 ) ;
#13944=CARTESIAN_POINT ( 'NONE',  ( 9.189545401991395579, 24.96013318841451678, 101.0000000000000000 ) ) ;
#13946=FACE_OUTER_BOUND ( 'NONE', #8308, .T. ) ;
#13947=DIRECTION ( 'NONE',  ( 1.000000000000000000, 0.000000000000000000, 0.000000000000000000 ) ) ;
#13950=CARTESIAN_POINT ( 'NONE',  ( 9.500222237632415911, 22.00424054664152607, 101.0000000000000000 ) ) ;
#13952=AXIS2_PLACEMENT_3D ( 'NONE', #6582, #14114, #5261 ) ;
#13960=AXIS2_PLACEMENT_3D ( 'NONE', #10524, #9275, #8095 ) ;
#13963=VERTEX_POINT ( 'NONE', #1052 ) ;
#13982=CIRCLE ( 'NONE', #9473, 17.50000000000000000 ) ;
#13983=CARTESIAN_POINT ( 'NONE',  ( -12.59082374547745076, 33.16401225666594854, 102.0000000000000142 ) ) ;
#13988=VERTEX_POINT ( 'NONE', #16024 ) ;
#13995=AXIS2_PLACEMENT_3D ( 'NONE', #14430, #6821, #14358 ) ;
#14007=ORIENTED_EDGE ( 'NONE', *, *, #9447, .F. ) ;
#14010=DIRECTION ( 'NONE',  ( -0.3090169943749448977, -0.9510565162951543083, 0.000000000000000000 ) ) ;
#14012=FACE_OUTER_BOUND ( 'NONE', #5640, .T. ) ;
#14028=ORIENTED_EDGE ( 'NONE', *, *, #4907, .T. ) ;
#14034=FACE_OUTER_BOUND ( 'NONE', #4126, .T. ) ;
#14076=CARTESIAN_POINT ( 'NONE',  ( 3.149380788944009968, 5.278461141749541063, 101.0000000000000000 ) ) ;
#14092=FACE_OUTER_BOUND ( 'NONE', #8236, .T. ) ;
#14093=FACE_OUTER_BOUND ( 'NONE', #6819, .T. ) ;
#14097=CARTESIAN_POINT ( 'NONE',  ( -10.69075041230567891, 8.636095224584611429, 102.0000000000000142 ) ) ;
#14108=VERTEX_POINT ( 'NONE', #3755 ) ;
#14109=ORIENTED_EDGE ( 'NONE', *, *, #9057, .F. ) ;
#14114=DIRECTION ( 'NONE',  ( 0.1045284632676435066, 0.9945218953682744001, 0.000000000000000000 ) ) ;
#14115=DIRECTION ( 'NONE',  ( 1.000000000000000000, 1.962715704248044508E-14, 0.000000000000000000 ) ) ;
#14117=DIRECTION ( 'NONE',  ( 0.1045284632676570929, -0.9945218953682730678, 0.000000000000000000 ) ) ;
#14127=EDGE_CURVE ( 'NONE', #8525, #10911, #11476, .T. ) ;
#14134=B_SPLINE_CURVE_WITH_KNOTS ( 'NONE', 3,
 ( #1836, #15646, #3008, #4350 ),
 .UNSPECIFIED., .F., .F.,
 ( 4, 4 ),
 ( 2.829004760677457000E-07, 0.001414802801989367004 ),
 .UNSPECIFIED. ) ;
#14136=PLANE ( 'NONE',  #2267 ) ;
#14139=DIRECTION ( 'NONE',  ( 0.4067366430758010964, -0.9135454576426004225, 0.000000000000000000 ) ) ;
#14148=VECTOR ( 'NONE', #13735, 1000.000000000000000 ) ;
#14151=VERTEX_POINT ( 'NONE', #6756 ) ;
#14153=EDGE_CURVE ( 'NONE', #10059, #3819, #10416, .T. ) ;
#14171=VERTEX_POINT ( 'NONE', #15539 ) ;
#14177=EDGE_CURVE ( 'NONE', #14691, #14171, #7981, .T. ) ;
#14179=DIRECTION ( 'NONE',  ( 0.000000000000000000, 0.000000000000000000, -1.000000000000000000 ) ) ;
#14193=FACE_OUTER_BOUND ( 'NONE', #9248, .T. ) ;
#14201=CARTESIAN_POINT ( 'NONE',  ( -13.33959974903384627, 33.83821319854129683, 101.0000000000000000 ) ) ;
#14206=ORIENTED_EDGE ( 'NONE', *, *, #3362, .F. ) ;
#14210=AXIS2_PLACEMENT_3D ( 'NONE', #15099, #3726, #8785 ) ;
#14211=DIRECTION ( 'NONE',  ( -0.3090169943749573878, 0.9510565162951503115, 0.000000000000000000 ) ) ;
#14217=DIRECTION ( 'NONE',  ( -1.000000000000000000, 0.000000000000000000, 0.000000000000000000 ) ) ;
#14226=AXIS2_PLACEMENT_3D ( 'NONE', #5252, #15518, #2898 ) ;
#14233=DIRECTION ( 'NONE',  ( 0.9781476007338069101, -0.2079116908177532363, 0.000000000000000000 ) ) ;
#14238=ORIENTED_EDGE ( 'NONE', *, *, #9780, .T. ) ;
#14243=AXIS2_PLACEMENT_3D ( 'NONE', #11573, #3771, #11260 ) ;
#14244=CARTESIAN_POINT ( 'NONE',  ( 9.877534094663406705, 8.054089844915898411, 101.0000000000000000 ) ) ;
#14247=DIRECTION ( 'NONE',  ( 0.000000000000000000, 0.000000000000000000, 1.000000000000000000 ) ) ;
#14256=CARTESIAN_POINT ( 'NONE',  ( 16.68146630878714731, 20.24395310072318921, 101.6666710451724214 ) ) ;
#14261=CARTESIAN_POINT ( 'NONE',  ( 14.53285685708578256, 14.68680145065703080, 102.0000000000000142 ) ) ;
#14270=DIRECTION ( 'NONE',  ( 0.5000000000000039968, -0.8660254037844363761, 0.000000000000000000 ) ) ;
#14273=VECTOR ( 'NONE', #3142, 1000.000000000000000 ) ;
#14285=DIRECTION ( 'NONE',  ( -0.000000000000000000, -0.000000000000000000, 1.000000000000000000 ) ) ;
#14287=VECTOR ( 'NONE', #13628, 1000.000000000000000 ) ;
#14301=EDGE_LOOP ( 'NONE', ( #12854, #875, #14109, #2540 ) ) ;
#14304=DIRECTION ( 'NONE',  ( -0.5877852522924797984, 0.8090169943749424553, 0.000000000000000000 ) ) ;
#14313=AXIS2_PLACEMENT_3D ( 'NONE', #9387, #14437, #9628 ) ;
#14320=ADVANCED_FACE ( 'NONE', ( #9633 ), #8470, .F. ) ;
#14325=FACE_OUTER_BOUND ( 'NONE', #15094, .T. ) ;
#14330=PLANE ( 'NONE',  #12364 ) ;
#14337=ORIENTED_EDGE ( 'NONE', *, *, #11252, .F. ) ;
#14343=EDGE_CURVE ( 'NONE', #7423, #11991, #4681, .T. ) ;
#14347=FACE_OUTER_BOUND ( 'NONE', #6344, .T. ) ;
#14352=DIRECTION ( 'NONE',  ( 0.000000000000000000, 0.000000000000000000, -1.000000000000000000 ) ) ;
#14358=DIRECTION ( 'NONE',  ( -0.9510565162951503115, -0.3090169943749574988, 0.000000000000000000 ) ) ;
#14364=CARTESIAN_POINT ( 'NONE',  ( 0.5000000000000000000, 39.99285568453590400, 101.0000000000000000 ) ) ;
#14376=LINE ( 'NONE', #15881, #4438 ) ;
#14378=VERTEX_POINT ( 'NONE', #8148 ) ;
#14390=CARTESIAN_POINT ( 'NONE',  ( 0.000000000000000000, 22.50000000000000000, 102.0000000000000142 ) ) ;
#14394=ORIENTED_EDGE ( 'NONE', *, *, #8730, .T. ) ;
#14414=DIRECTION ( 'NONE',  ( 1.000000000000000000, -1.784287003861858895E-15, 0.000000000000000000 ) ) ;
#14423=EDGE_CURVE ( 'NONE', #589, #13963, #15725, .T. ) ;
#14426=ORIENTED_EDGE ( 'NONE', *, *, #3820, .F. ) ;
#14428=VERTEX_POINT ( 'NONE', #4656 ) ;
#14429=ORIENTED_EDGE ( 'NONE', *, *, #1841, .F. ) ;
#14430=CARTESIAN_POINT ( 'NONE',  ( 16.79799753235259985, 27.43226914341417810, 101.0000000000000000 ) ) ;
#14431=DIRECTION ( 'NONE',  ( 0.000000000000000000, 0.000000000000000000, 1.000000000000000000 ) ) ;
#14437=DIRECTION ( 'NONE',  ( 0.000000000000000000, 0.000000000000000000, 1.000000000000000000 ) ) ;
#14448=ORIENTED_EDGE ( 'NONE', *, *, #1221, .F. ) ;
#14452=ORIENTED_EDGE ( 'NONE', *, *, #1873, .F. ) ;
#14475=AXIS2_PLACEMENT_3D ( 'NONE', #9834, #3513, #2164 ) ;
#14479=VECTOR ( 'NONE', #15304, 1000.000000000000000 ) ;
#14492=AXIS2_PLACEMENT_3D ( 'NONE', #107, #13831, #3867 ) ;
#14497=CARTESIAN_POINT ( 'NONE',  ( 3.149380788944009968, 5.278461141749541063, 101.0000000000000000 ) ) ;
#14501=CARTESIAN_POINT ( 'NONE',  ( 14.90544456622775904, 13.31698729810792692, 101.0000000000000000 ) ) ;
#14510=VERTEX_POINT ( 'NONE', #3229 ) ;
#14511=EDGE_CURVE ( 'NONE', #7047, #14534, #9725, .T. ) ;
#14513=ORIENTED_EDGE ( 'NONE', *, *, #2957, .F. ) ;
#14514=ORIENTED_EDGE ( 'NONE', *, *, #5256, .F. ) ;
#14519=LINE ( 'NONE', #13361, #14273 ) ;
#14525=ADVANCED_FACE ( 'NONE', ( #13856 ), #13695, .F. ) ;
#14527=DIRECTION ( 'NONE',  ( 1.224646799147353207E-16, -1.000000000000000000, 0.000000000000000000 ) ) ;
#14531=EDGE_CURVE ( 'NONE', #11153, #3858, #6982, .T. ) ;
#14534=VERTEX_POINT ( 'NONE', #6075 ) ;
#14539=ORIENTED_EDGE ( 'NONE', *, *, #1354, .T. ) ;
#14549=FACE_OUTER_BOUND ( 'NONE', #9617, .T. ) ;
#14558=ORIENTED_EDGE ( 'NONE', *, *, #10918, .F. ) ;
#14559=FACE_OUTER_BOUND ( 'NONE', #7348, .T. ) ;
#14575=VERTEX_POINT ( 'NONE', #10052 ) ;
#14591=APPLICATION_CONTEXT ( 'automotive_design' ) ;
#14595=DIRECTION ( 'NONE',  ( -0.8660254037844433705, 0.4999999999999918954, 0.000000000000000000 ) ) ;
#14598=DIRECTION ( 'NONE',  ( 0.1045284632676435066, 0.9945218953682744001, 0.000000000000000000 ) ) ;
#14601=CARTESIAN_POINT ( 'NONE',  ( -3.407225380398804404, 31.38205016914259105, 101.0000000000000000 ) ) ;
#14604=CARTESIAN_POINT ( 'NONE',  ( 0.5000000000000000000, 39.99999999999999289, 101.0000000000000000 ) ) ;
#14612=ORIENTED_EDGE ( 'NONE', *, *, #12442, .F. ) ;
#14615=CARTESIAN_POINT ( 'NONE',  ( 17.50000000000000000, 22.50000000000000355, 102.0000000000000142 ) ) ;
#14622=EDGE_CURVE ( 'NONE', #860, #10405, #8792, .T. ) ;
#14627=DIRECTION ( 'NONE',  ( 0.2079116908177531253, 0.9781476007338069101, 0.000000000000000000 ) ) ;
#14633=VERTEX_POINT ( 'NONE', #9047 ) ;
#14655=ORIENTED_EDGE ( 'NONE', *, *, #6067, .F. ) ;
#14666=VECTOR ( 'NONE', #14304, 1000.000000000000227 ) ;
#14668=VERTEX_POINT ( 'NONE', #1635 ) ;
#14670=EDGE_CURVE ( 'NONE', #5931, #15550, #7247, .T. ) ;
#14671=VERTEX_POINT ( 'NONE', #12704 ) ;
#14674=B_SPLINE_CURVE_WITH_KNOTS ( 'NONE', 3,
 ( #7732, #12799, #15124, #6493 ),
 .UNSPECIFIED., .F., .F.,
 ( 4, 4 ),
 ( 2.829004760683498992E-07, 0.001414802801989366787 ),
 .UNSPECIFIED. ) ;
#14682=DIRECTION ( 'NONE',  ( 0.000000000000000000, -1.000000000000000000, 0.000000000000000000 ) ) ;
#14688=EDGE_LOOP ( 'NONE', ( #2188, #8517, #16448, #9013 ) ) ;
#14691=VERTEX_POINT ( 'NONE', #15435 ) ;
#14693=VECTOR ( 'NONE', #9334, 1000.000000000000000 ) ;
#14694=VECTOR ( 'NONE', #13796, 1000.000000000000000 ) ;
#14711=EDGE_CURVE ( 'NONE', #7047, #11303, #6730, .T. ) ;
#14718=CARTESIAN_POINT ( 'NONE',  ( 10.69075041230586365, 8.636095224584757091, 101.0000000000000000 ) ) ;
#14720=ADVANCED_FACE ( 'NONE', ( #1558 ), #6652, .F. ) ;
#14726=CARTESIAN_POINT ( 'NONE',  ( 15.39925740754319605, 14.18658485962441240, 101.0000000000000000 ) ) ;
#14727=EDGE_CURVE ( 'NONE', #8593, #12133, #10458, .T. ) ;
#14730=AXIS2_PLACEMENT_3D ( 'NONE', #4484, #14847, #14595 ) ;
#14738=VECTOR ( 'NONE', #11524, 1000.000000000000114 ) ;
#14739=CIRCLE ( 'NONE', #9444, 7.732050807568878525 ) ;
#14762=CARTESIAN_POINT ( 'NONE',  ( 0.000000000000000000, 22.50000000000000000, 100.0000000000000000 ) ) ;
#14772=CARTESIAN_POINT ( 'NONE',  ( 12.66515988160610107, 34.57657754388035443, 101.0000000000000000 ) ) ;
#14775=ORIENTED_EDGE ( 'NONE', *, *, #5200, .F. ) ;
#14780=AXIS2_PLACEMENT_3D ( 'NONE', #5257, #16371, #16455 ) ;
#14783=DIRECTION ( 'NONE',  ( -0.000000000000000000, -0.000000000000000000, -1.000000000000000000 ) ) ;
#14784=ORIENTED_EDGE ( 'NONE', *, *, #14531, .T. ) ;
#14787=AXIS2_PLACEMENT_3D ( 'NONE', #769, #5859, #13491 ) ;
#14804=CARTESIAN_POINT ( 'NONE',  ( 9.500222237632415911, 22.00424054664152607, 102.0000000000000142 ) ) ;
#14809=DIRECTION ( 'NONE',  ( -0.3090169943749448977, -0.9510565162951543083, 0.000000000000000000 ) ) ;
#14826=CONICAL_SURFACE ( 'NONE', #7677, 16.50000000000000711, 0.7853981633974447263 ) ;
#14840=EDGE_CURVE ( 'NONE', #2743, #860, #11758, .T. ) ;
#14847=DIRECTION ( 'NONE',  ( 0.4999999999999918954, 0.8660254037844433705, 0.000000000000000000 ) ) ;
#14851=VECTOR ( 'NONE', #1396, 1000.000000000000000 ) ;
#14855=DIRECTION ( 'NONE',  ( -0.8660254037844433705, 0.4999999999999918399, 0.000000000000000000 ) ) ;
#14857=DIRECTION ( 'NONE',  ( 1.000000000000000000, 0.000000000000000000, 0.000000000000000000 ) ) ;
#14860=ORIENTED_EDGE ( 'NONE', *, *, #10152, .F. ) ;
#14869=ORIENTED_EDGE ( 'NONE', *, *, #6070, .F. ) ;
#14871=CARTESIAN_POINT ( 'NONE',  ( 4.678013043399448456, 44.50832101651065642, 101.0000000000000000 ) ) ;
#14875=DIRECTION ( 'NONE',  ( 0.5877852522924797984, -0.8090169943749426773, 0.000000000000000000 ) ) ;
#14892=EDGE_CURVE ( 'NONE', #12041, #5661, #792, .T. ) ;
#14893=DIRECTION ( 'NONE',  ( -0.5877852522924797984, 0.8090169943749424553, 0.000000000000000000 ) ) ;
#14894=CARTESIAN_POINT ( 'NONE',  ( 0.000000000000000000, 22.50000000000000000, 101.0000000000000000 ) ) ;
#14918=ORIENTED_EDGE ( 'NONE', *, *, #14622, .T. ) ;
#14925=ORIENTED_EDGE ( 'NONE', *, *, #12723, .T. ) ;
#14926=PLANE ( 'NONE',  #4730 ) ;
#14935=DIRECTION ( 'NONE',  ( 0.000000000000000000, 0.000000000000000000, 1.000000000000000000 ) ) ;
#14944=LINE ( 'NONE', #13803, #2277 ) ;
#14952=ORIENTED_EDGE ( 'NONE', *, *, #210, .T. ) ;
#14954=( NAMED_UNIT ( * ) SI_UNIT ( $, .STERADIAN. ) SOLID_ANGLE_UNIT ( ) );
#14955=CARTESIAN_POINT ( 'NONE',  ( -3.149380788943775933, 5.278461141749506425, 101.0000000000000000 ) ) ;
#14959=CARTESIAN_POINT ( 'NONE',  ( 0.5000000000000001110, 39.32590460608501104, 101.6666710454654208 ) ) ;
#14963=CARTESIAN_POINT ( 'NONE',  ( 6.658212670116058440, 38.68388717334331517, 101.0000000000000000 ) ) ;
#14966=DIRECTION ( 'NONE',  ( 0.000000000000000000, 0.000000000000000000, 1.000000000000000000 ) ) ;
#14971=ORIENTED_EDGE ( 'NONE', *, *, #5117, .T. ) ;
#14975=FACE_OUTER_BOUND ( 'NONE', #11730, .T. ) ;
#14981=DIRECTION ( 'NONE',  ( -0.9135454576426060846, 0.4067366430757887730, 0.000000000000000000 ) ) ;
#15009=ORIENTED_EDGE ( 'NONE', *, *, #11413, .T. ) ;
#15012=EDGE_CURVE ( 'NONE', #1326, #15748, #2855, .T. ) ;
#15014=PLANE ( 'NONE',  #2617 ) ;
#15022=DIRECTION ( 'NONE',  ( -1.000000000000000000, 0.000000000000000000, 0.000000000000000000 ) ) ;
#15023=VECTOR ( 'NONE', #1398, 1000.000000000000000 ) ;
#15029=EDGE_CURVE ( 'NONE', #7317, #13034, #6779, .T. ) ;
#15036=VECTOR ( 'NONE', #10084, 1000.000000000000227 ) ;
#15051=VECTOR ( 'NONE', #7695, 1000.000000000000000 ) ;
#15052=DIRECTION ( 'NONE',  ( 1.000000000000000000, 0.000000000000000000, 0.000000000000000000 ) ) ;
#15061=ADVANCED_FACE ( 'NONE', ( #1601 ), #6695, .T. ) ;
#15068=DIRECTION ( 'NONE',  ( 0.9781476007338042455, 0.2079116908177664758, 0.000000000000000000 ) ) ;
#15092=AXIS2_PLACEMENT_3D ( 'NONE', #7484, #10315, #14117 ) ;
#15094=EDGE_LOOP ( 'NONE', ( #323, #941, #1276, #9727 ) ) ;
#15099=CARTESIAN_POINT ( 'NONE',  ( 10.69075041230586365, 8.636095224584757091, 101.0000000000000000 ) ) ;
#15100=DIRECTION ( 'NONE',  ( 0.1045284632676570929, -0.9945218953682730678, 0.000000000000000000 ) ) ;
#15108=ORIENTED_EDGE ( 'NONE', *, *, #9318, .F. ) ;
#15117=CARTESIAN_POINT ( 'NONE',  ( 8.477241335952196977, 18.18301270189230578, 101.0000000000000000 ) ) ;
#15124=CARTESIAN_POINT ( 'NONE',  ( 10.29452708129665162, 9.181449853854692478, 101.6666710451724214 ) ) ;
#15126=CARTESIAN_POINT ( 'NONE',  ( 6.522576737113721101, 38.37924387995723663, 101.3333374614808662 ) ) ;
#15135=EDGE_CURVE ( 'NONE', #15748, #1641, #10671, .T. ) ;
#15143=FACE_OUTER_BOUND ( 'NONE', #3818, .T. ) ;
#15147=EDGE_CURVE ( 'NONE', #2544, #1479, #674, .T. ) ;
#15151=ADVANCED_FACE ( 'NONE', ( #3099 ), #8039, .T. ) ;
#15155=ORIENTED_EDGE ( 'NONE', *, *, #7444, .F. ) ;
#15161=CARTESIAN_POINT ( 'NONE',  ( -3.147895402235901141, 5.285449336779595164, 101.0000000000000000 ) ) ;
#15170=EDGE_CURVE ( 'NONE', #286, #11447, #16148, .T. ) ;
#15173=EDGE_LOOP ( 'NONE', ( #6464, #4007, #10511, #11350 ) ) ;
#15183=VERTEX_POINT ( 'NONE', #12315 ) ;
#15184=EDGE_CURVE ( 'NONE', #12542, #13034, #13315, .T. ) ;
#15185=VECTOR ( 'NONE', #8304, 1000.000000000000000 ) ;
#15187=EDGE_CURVE ( 'NONE', #8086, #14691, #12023, .T. ) ;
#15193=DIRECTION ( 'NONE',  ( 1.000000000000000000, 0.000000000000000000, 0.000000000000000000 ) ) ;
#15194=DIRECTION ( 'NONE',  ( 0.000000000000000000, 0.000000000000000000, 1.000000000000000000 ) ) ;
#15198=LINE ( 'NONE', #1319, #15898 ) ;
#15211=DIRECTION ( 'NONE',  ( 1.224646799147353207E-16, -1.000000000000000000, 0.000000000000000000 ) ) ;
#15245=CARTESIAN_POINT ( 'NONE',  ( -13.08647130699031713, 33.61029532559849287, 101.3333374614808662 ) ) ;
#15254=CARTESIAN_POINT ( 'NONE',  ( -0.5000000000000000000, 39.99285568453590400, 101.0000000000000000 ) ) ;
#15255=DIRECTION ( 'NONE',  ( 1.000000000000000000, 0.000000000000000000, 0.000000000000000000 ) ) ;
#15269=ORIENTED_EDGE ( 'NONE', *, *, #8476, .F. ) ;
#15273=AXIS2_PLACEMENT_3D ( 'NONE', #12001, #3024, #2869 ) ;
#15279=CARTESIAN_POINT ( 'NONE',  ( -17.34476375915448187, 20.17423772944842142, 101.0000000000000000 ) ) ;
#15281=AXIS2_PLACEMENT_3D ( 'NONE', #702, #4545, #7124 ) ;
#15298=AXIS2_PLACEMENT_3D ( 'NONE', #10567, #6748, #10807 ) ;
#15304=DIRECTION ( 'NONE',  ( 0.5877852522924688072, 0.8090169943749505599, 0.000000000000000000 ) ) ;
#15324=ORIENTED_EDGE ( 'NONE', *, *, #10540, .F. ) ;
#15337=APPLICATION_CONTEXT ( 'automotive_design' ) ;
#15341=EDGE_LOOP ( 'NONE', ( #13063, #10914, #10183, #4412 ) ) ;
#15344=CARTESIAN_POINT ( 'NONE',  ( -12.41734070063146156, 34.35344015107588689, 101.3333374614808662 ) ) ;
#15353=LINE ( 'NONE', #9122, #5180 ) ;
#15360=ORIENTED_EDGE ( 'NONE', *, *, #2912, .T. ) ;
#15362=ORIENTED_EDGE ( 'NONE', *, *, #13064, .T. ) ;
#15366=DIRECTION ( 'NONE',  ( -0.9135454576426059736, 0.4067366430757887730, 0.000000000000000000 ) ) ;
#15371=SHAPE_REPRESENTATION_RELATIONSHIP ( 'NONE' , 'NONE' ,  #13393, #12174 ) ;
#15381=( GEOMETRIC_REPRESENTATION_CONTEXT ( 3 ) GLOBAL_UNCERTAINTY_ASSIGNED_CONTEXT ( ( #4441 ) ) GLOBAL_UNIT_ASSIGNED_CONTEXT ( ( #7325, #987, #14954 ) ) REPRESENTATION_CONTEXT ( 'NONE', 'WORKASPACE' ) );
#15393=CIRCLE ( 'NONE', #13004, 16.50000000000000711 ) ;
#15395=DIRECTION ( 'NONE',  ( 0.000000000000000000, 0.000000000000000000, -1.000000000000000000 ) ) ;
#15400=EDGE_CURVE ( 'NONE', #14510, #562, #926, .T. ) ;
#15408=VERTEX_POINT ( 'NONE', #12740 ) ;
#15429=CARTESIAN_POINT ( 'NONE',  ( 0.5000000000000000000, 39.99285568453590400, 101.0000000000000000 ) ) ;
#15430=LINE ( 'NONE', #14097, #11150 ) ;
#15435=CARTESIAN_POINT ( 'NONE',  ( -17.44929222242214095, 21.16875962481669760, 101.0000000000000000 ) ) ;
#15436=ORIENTED_EDGE ( 'NONE', *, *, #11589, .F. ) ;
#15442=EDGE_LOOP ( 'NONE', ( #7446, #414, #11854, #3857 ) ) ;
#15452=EDGE_CURVE ( 'NONE', #2396, #5969, #2752, .T. ) ;
#15453=PLANE ( 'NONE',  #8337 ) ;
#15459=EDGE_CURVE ( 'NONE', #4499, #895, #11900, .T. ) ;
#15461=ORIENTED_EDGE ( 'NONE', *, *, #6958, .T. ) ;
#15469=DIRECTION ( 'NONE',  ( -0.4067366430757887175, -0.9135454576426059736, 0.000000000000000000 ) ) ;
#15479=VECTOR ( 'NONE', #9835, 1000.000000000000000 ) ;
#15487=DIRECTION ( 'NONE',  ( 0.000000000000000000, 0.000000000000000000, 1.000000000000000000 ) ) ;
#15489=VECTOR ( 'NONE', #65, 999.9999999999998863 ) ;
#15492=CARTESIAN_POINT ( 'NONE',  ( 5.179451399591075145, 14.52044592729181538, 102.0000000000000142 ) ) ;
#15498=AXIS2_PLACEMENT_3D ( 'NONE', #3994, #1495, #238 ) ;
#15500=ORIENTED_EDGE ( 'NONE', *, *, #711, .T. ) ;
#15515=ORIENTED_EDGE ( 'NONE', *, *, #15452, .T. ) ;
#15518=DIRECTION ( 'NONE',  ( 0.7431448254773862505, 0.6691306063588672304, 0.000000000000000000 ) ) ;
#15525=PLANE ( 'NONE',  #12082 ) ;
#15529=CARTESIAN_POINT ( 'NONE',  ( 0.000000000000000000, 22.50000000000000000, 102.0000000000000142 ) ) ;
#15539=CARTESIAN_POINT ( 'NONE',  ( -9.500222237632405253, 22.00424054664139817, 101.0000000000000000 ) ) ;
#15540=ADVANCED_FACE ( 'NONE', ( #15713 ), #7259, .T. ) ;
#15543=ORIENTED_EDGE ( 'NONE', *, *, #3052, .T. ) ;
#15544=ORIENTED_EDGE ( 'NONE', *, *, #10785, .F. ) ;
#15547=CARTESIAN_POINT ( 'NONE',  ( -0.5000000000000000000, 39.99999999999999289, 101.0000000000000000 ) ) ;
#15549=AXIS2_PLACEMENT_3D ( 'NONE', #2347, #1168, #11255 ) ;
#15550=VERTEX_POINT ( 'NONE', #254 ) ;
#15551=PRODUCT_DEFINITION_SHAPE ( 'NONE', 'NONE',  #2740 ) ;
#15563=AXIS2_PLACEMENT_3D ( 'NONE', #16223, #14966, #15052 ) ;
#15569=EDGE_CURVE ( 'NONE', #960, #7551, #10736, .T. ) ;
#15590=EDGE_CURVE ( 'NONE', #15550, #6081, #1511, .T. ) ;
#15591=VECTOR ( 'NONE', #9797, 1000.000000000000000 ) ;
#15597=ORIENTED_EDGE ( 'NONE', *, *, #10903, .T. ) ;
#15598=DIRECTION ( 'NONE',  ( 0.5000000000000041078, -0.8660254037844363761, -0.000000000000000000 ) ) ;
#15600=CARTESIAN_POINT ( 'NONE',  ( 4.056709942754594067, 5.819547430268785959, 101.3333374614808662 ) ) ;
#15603=DIRECTION ( 'NONE',  ( 0.000000000000000000, 0.000000000000000000, 1.000000000000000000 ) ) ;
#15619=CARTESIAN_POINT ( 'NONE',  ( 0.5000000000000009992, 31.99999999999998579, 101.0000000000000000 ) ) ;
#15621=VECTOR ( 'NONE', #6142, 1000.000000000000227 ) ;
#15625=CARTESIAN_POINT ( 'NONE',  ( -16.47405064338592595, 27.32701241865528985, 101.3333374614808662 ) ) ;
#15630=ORIENTED_EDGE ( 'NONE', *, *, #4081, .T. ) ;
#15631=EDGE_LOOP ( 'NONE', ( #15436, #5296, #9857, #16205 ) ) ;
#15638=PLANE ( 'NONE',  #1744 ) ;
#15640=CARTESIAN_POINT ( 'NONE',  ( -4.127528389677584286, 5.486372832567261604, 102.0000000000000142 ) ) ;
#15646=CARTESIAN_POINT ( 'NONE',  ( 3.078562342020788822, 5.611635739451020122, 101.3333374614808662 ) ) ;
#15650=DIRECTION ( 'NONE',  ( 0.000000000000000000, 0.000000000000000000, -1.000000000000000000 ) ) ;
#15652=EDGE_CURVE ( 'NONE', #1083, #6085, #11656, .T. ) ;
#15658=DIRECTION ( 'NONE',  ( 1.000000000000000000, -6.145877457746401939E-15, 0.000000000000000000 ) ) ;
#15667=EDGE_CURVE ( 'NONE', #13340, #605, #9916, .T. ) ;
#15672=VERTEX_POINT ( 'NONE', #5521 ) ;
#15697=CARTESIAN_POINT ( 'NONE',  ( -10.29452708129647220, 9.181449853854553922, 101.6666710451724214 ) ) ;
#15706=ORIENTED_EDGE ( 'NONE', *, *, #14622, .F. ) ;
#15710=EDGE_LOOP ( 'NONE', ( #12866, #12273, #7071, #5907 ) ) ;
#15713=FACE_OUTER_BOUND ( 'NONE', #11173, .T. ) ;
#15725=CIRCLE ( 'NONE', #5401, 16.50000000000000711 ) ;
#15737=VECTOR ( 'NONE', #9755, 999.9999999999998863 ) ;
#15742=EDGE_CURVE ( 'NONE', #3406, #3901, #9823, .T. ) ;
#15748=VERTEX_POINT ( 'NONE', #12054 ) ;
#15758=VECTOR ( 'NONE', #5673, 1000.000000000000000 ) ;
#15774=DIRECTION ( 'NONE',  ( 0.9781476007338069101, -0.2079116908177532363, 0.000000000000000000 ) ) ;
#15784=CONICAL_SURFACE ( 'NONE', #1451, 16.50000000000000711, 0.7853981633974447263 ) ;
#15787=ORIENTED_EDGE ( 'NONE', *, *, #7266, .T. ) ;
#15791=LINE ( 'NONE', #11972, #6298 ) ;
#15794=CARTESIAN_POINT ( 'NONE',  ( -3.987376076617207499, 6.145737624504182151, 101.6666710451724214 ) ) ;
#15795=DIRECTION ( 'NONE',  ( 1.000000000000000000, 0.000000000000000000, -0.000000000000000000 ) ) ;
#15796=CARTESIAN_POINT ( 'NONE',  ( 0.000000000000000000, 22.50000000000000000, 102.0000000000000142 ) ) ;
#15798=VECTOR ( 'NONE', #6140, 1000.000000000000000 ) ;
#15809=VECTOR ( 'NONE', #10087, 1000.000000000000000 ) ;
#15811=ORIENTED_EDGE ( 'NONE', *, *, #7941, .T. ) ;
#15812=AXIS2_PLACEMENT_3D ( 'NONE', #2158, #11073, #8560 ) ;
#15820=AXIS2_PLACEMENT_3D ( 'NONE', #9858, #13667, #7373 ) ;
#15837=AXIS2_PLACEMENT_3D ( 'NONE', #9804, #14682, #13773 ) ;
#15840=ORIENTED_EDGE ( 'NONE', *, *, #7249, .F. ) ;
#15842=CARTESIAN_POINT ( 'NONE',  ( -16.48898053797772789, 28.38332565970911148, 101.0000000000000000 ) ) ;
#15847=DIRECTION ( 'NONE',  ( -1.000000000000000000, 0.000000000000000000, 0.000000000000000000 ) ) ;
#15848=AXIS2_PLACEMENT_3D ( 'NONE', #15970, #6495, #12559 ) ;
#15851=CONICAL_SURFACE ( 'NONE', #14780, 16.50000000000000711, 0.7853981633974447263 ) ;
#15861=CARTESIAN_POINT ( 'NONE',  ( 16.16503364901090123, 28.27806893495066021, 101.3333374614808662 ) ) ;
#15878=ORIENTED_EDGE ( 'NONE', *, *, #9988, .F. ) ;
#15881=CARTESIAN_POINT ( 'NONE',  ( 9.189545401991395579, 24.96013318841451678, 102.0000000000000142 ) ) ;
#15884=CARTESIAN_POINT ( 'NONE',  ( 0.000000000000000000, 22.50000000000000000, 100.0000000000000000 ) ) ;
#15898=VECTOR ( 'NONE', #16462, 1000.000000000000000 ) ;
#15916=EDGE_CURVE ( 'NONE', #4820, #4055, #7652, .T. ) ;
#15920=ORIENTED_EDGE ( 'NONE', *, *, #9277, .T. ) ;
#15923=PLANE ( 'NONE',  #15281 ) ;
#15926=LINE ( 'NONE', #14501, #5189 ) ;
#15934=ORIENTED_EDGE ( 'NONE', *, *, #4622, .F. ) ;
#15935=ORIENTED_EDGE ( 'NONE', *, *, #4107, .F. ) ;
#15938=CARTESIAN_POINT ( 'NONE',  ( 12.41734070063129813, 34.35344015107605742, 101.3333374614808662 ) ) ;
#15961=ADVANCED_FACE ( 'NONE', ( #6408 ), #8892, .F. ) ;
#15967=CARTESIAN_POINT ( 'NONE',  ( -9.395693774364753281, 21.00971865127312199, 101.0000000000000000 ) ) ;
#15970=CARTESIAN_POINT ( 'NONE',  ( 7.574663982647604321, 38.28367718720770796, 101.0000000000000000 ) ) ;
#15977=ORIENTED_EDGE ( 'NONE', *, *, #5460, .T. ) ;
#15978=DIRECTION ( 'NONE',  ( -1.000000000000000000, 0.000000000000000000, 0.000000000000000000 ) ) ;
#15997=ORIENTED_EDGE ( 'NONE', *, *, #16301, .T. ) ;
#16024=CARTESIAN_POINT ( 'NONE',  ( 14.03285685708579145, 13.82077604687259154, 102.0000000000000142 ) ) ;
#16026=CARTESIAN_POINT ( 'NONE',  ( 12.67046914267482016, 34.58135802401886139, 101.0000000000000000 ) ) ;
#16037=CARTESIAN_POINT ( 'NONE',  ( 10.09851121871635904, 9.451242543235769844, 102.0000000000000142 ) ) ;
#16046=( NAMED_UNIT ( * ) PLANE_ANGLE_UNIT ( ) SI_UNIT ( $, .RADIAN. ) );
#16050=CARTESIAN_POINT ( 'NONE',  ( -3.149380788943775933, 5.278461141749506425, 101.0000000000000000 ) ) ;
#16051=VECTOR ( 'NONE', #2322, 1000.000000000000000 ) ;
#16055=CARTESIAN_POINT ( 'NONE',  ( 5.179451399591075145, 14.52044592729181538, 101.0000000000000000 ) ) ;
#16075=EDGE_CURVE ( 'NONE', #10305, #8817, #4624, .T. ) ;
#16077=( GEOMETRIC_REPRESENTATION_CONTEXT ( 3 ) GLOBAL_UNCERTAINTY_ASSIGNED_CONTEXT ( ( #4601 ) ) GLOBAL_UNIT_ASSIGNED_CONTEXT ( ( #8405, #16046, #3426 ) ) REPRESENTATION_CONTEXT ( 'NONE', 'WORKASPACE' ) );
#16082=ORIENTED_EDGE ( 'NONE', *, *, #10903, .F. ) ;
#16097=AXIS2_PLACEMENT_3D ( 'NONE', #7572, #1246, #11169 ) ;
#16099=CIRCLE ( 'NONE', #9469, 2.267949192431125027 ) ;
#16106=ORIENTED_EDGE ( 'NONE', *, *, #7347, .F. ) ;
#16115=CARTESIAN_POINT ( 'NONE',  ( -0.4999999999999990563, 31.99999999999998579, 102.0000000000000142 ) ) ;
#16120=DIRECTION ( 'NONE',  ( 0.4067366430758010964, -0.9135454576426004225, 0.000000000000000000 ) ) ;
#16123=ORIENTED_EDGE ( 'NONE', *, *, #2785, .F. ) ;
#16128=ORIENTED_EDGE ( 'NONE', *, *, #3960, .T. ) ;
#16136=CARTESIAN_POINT ( 'NONE',  ( -13.33429048796512717, 33.83343271840278277, 101.0000000000000000 ) ) ;
#16137=DIRECTION ( 'NONE',  ( -0.6691306063588569053, -0.7431448254773954654, 0.000000000000000000 ) ) ;
#16142=FACE_OUTER_BOUND ( 'NONE', #4253, .T. ) ;
#16144=DIRECTION ( 'NONE',  ( 0.000000000000000000, 0.000000000000000000, 1.000000000000000000 ) ) ;
#16147=DIRECTION ( 'NONE',  ( -0.9510565162951503115, -0.3090169943749574988, 0.000000000000000000 ) ) ;
#16148=LINE ( 'NONE', #16055, #15737 ) ;
#16152=DIRECTION ( 'NONE',  ( 0.000000000000000000, 0.000000000000000000, -1.000000000000000000 ) ) ;
#16155=DIRECTION ( 'NONE',  ( 0.9510565162951544194, -0.3090169943749448422, 0.000000000000000000 ) ) ;
#16163=AXIS2_PLACEMENT_3D ( 'NONE', #6163, #8557, #2079 ) ;
#16173=EDGE_CURVE ( 'NONE', #895, #1641, #12204, .T. ) ;
#16174=ORIENTED_EDGE ( 'NONE', *, *, #1271, .T. ) ;
#16202=VERTEX_POINT ( 'NONE', #5811 ) ;
#16204=EDGE_LOOP ( 'NONE', ( #900, #11805, #2685, #11208 ) ) ;
#16205=ORIENTED_EDGE ( 'NONE', *, *, #15012, .F. ) ;
#16212=DIRECTION ( 'NONE',  ( 0.9781476007338070211, -0.2079116908177531808, -0.000000000000000000 ) ) ;
#16215=CARTESIAN_POINT ( 'NONE',  ( 7.394441145214595501, 28.48516834767053751, 101.0000000000000000 ) ) ;
#16216=PLANE ( 'NONE',  #4174 ) ;
#16217=EDGE_CURVE ( 'NONE', #4275, #6384, #6978, .T. ) ;
#16220=FACE_OUTER_BOUND ( 'NONE', #9996, .T. ) ;
#16223=CARTESIAN_POINT ( 'NONE',  ( 0.000000000000000000, 22.50000000000000000, 100.0000000000000000 ) ) ;
#16231=CARTESIAN_POINT ( 'NONE',  ( 0.000000000000000000, 22.50000000000000000, 102.0000000000000142 ) ) ;
#16246=VERTEX_POINT ( 'NONE', #10500 ) ;
#16260=ORIENTED_EDGE ( 'NONE', *, *, #15184, .F. ) ;
#16275=VECTOR ( 'NONE', #4090, 1000.000000000000000 ) ;
#16276=CARTESIAN_POINT ( 'NONE',  ( 9.881733417930924190, 8.048309972292271297, 101.0000000000000000 ) ) ;
#16278=EDGE_CURVE ( 'NONE', #13988, #9739, #5362, .T. ) ;
#16280=EDGE_LOOP ( 'NONE', ( #13597, #4661, #11477, #3572 ) ) ;
#16282=ORIENTED_EDGE ( 'NONE', *, *, #2912, .F. ) ;
#16285=CARTESIAN_POINT ( 'NONE',  ( 7.436122194756328518, 37.97250723688144802, 101.3333374614808662 ) ) ;
#16286=EDGE_CURVE ( 'NONE', #12958, #7234, #10665, .T. ) ;
#16301=EDGE_CURVE ( 'NONE', #7423, #10059, #12297, .T. ) ;
#16302=DIRECTION ( 'NONE',  ( -0.7431448254773861395, -0.6691306063588672304, 0.000000000000000000 ) ) ;
#16305=EDGE_LOOP ( 'NONE', ( #6780, #5311 ) ) ;
#16307=ORIENTED_EDGE ( 'NONE', *, *, #5316, .T. ) ;
#16311=CARTESIAN_POINT ( 'NONE',  ( 8.880528407616436581, 25.91118970470966687, 102.0000000000000142 ) ) ;
#16314=AXIS2_PLACEMENT_3D ( 'NONE', #7607, #9021, #13751 ) ;
#16328=EDGE_LOOP ( 'NONE', ( #5143, #7300, #8456, #5026 ) ) ;
#16332=DIRECTION ( 'NONE',  ( 0.000000000000000000, 0.000000000000000000, -1.000000000000000000 ) ) ;
#16335=VECTOR ( 'NONE', #12609, 999.9999999999998863 ) ;
#16349=CARTESIAN_POINT ( 'NONE',  ( 9.395693774364776374, 21.00971865127324634, 101.0000000000000000 ) ) ;
#16356=VECTOR ( 'NONE', #3827, 1000.000000000000000 ) ;
#16368=AXIS2_PLACEMENT_3D ( 'NONE', #6269, #12666, #1264 ) ;
#16369=CONICAL_SURFACE ( 'NONE', #4718, 16.50000000000000711, 0.7853981633974447263 ) ;
#16371=DIRECTION ( 'NONE',  ( 0.000000000000000000, 0.000000000000000000, -1.000000000000000000 ) ) ;
#16378=CARTESIAN_POINT ( 'NONE',  ( -17.01311696148842501, 20.20909521249542706, 101.3333374614808662 ) ) ;
#16382=CARTESIAN_POINT ( 'NONE',  ( 2.464234863135679188, 13.31155363843775064, 101.0000000000000000 ) ) ;
#16396=ORIENTED_EDGE ( 'NONE', *, *, #7214, .T. ) ;
#16418=ORIENTED_EDGE ( 'NONE', *, *, #3535, .T. ) ;
#16423=FACE_OUTER_BOUND ( 'NONE', #3468, .T. ) ;
#16443=AXIS2_PLACEMENT_3D ( 'NONE', #14871, #13624, #6087 ) ;
#16446=PLANE ( 'NONE',  #3674 ) ;
#16448=ORIENTED_EDGE ( 'NONE', *, *, #10794, .F. ) ;
#16455=DIRECTION ( 'NONE',  ( -1.000000000000000000, 0.000000000000000000, 0.000000000000000000 ) ) ;
#16460=CARTESIAN_POINT ( 'NONE',  ( 0.000000000000000000, 22.50000000000000000, 101.0000000000000000 ) ) ;
#16462=DIRECTION ( 'NONE',  ( -0.6691306063588671194, 0.7431448254773862505, 0.000000000000000000 ) ) ;
#16463=( NAMED_UNIT ( * ) SI_UNIT ( $, .STERADIAN. ) SOLID_ANGLE_UNIT ( ) );
ENDSEC;
END-ISO-10303-21;
